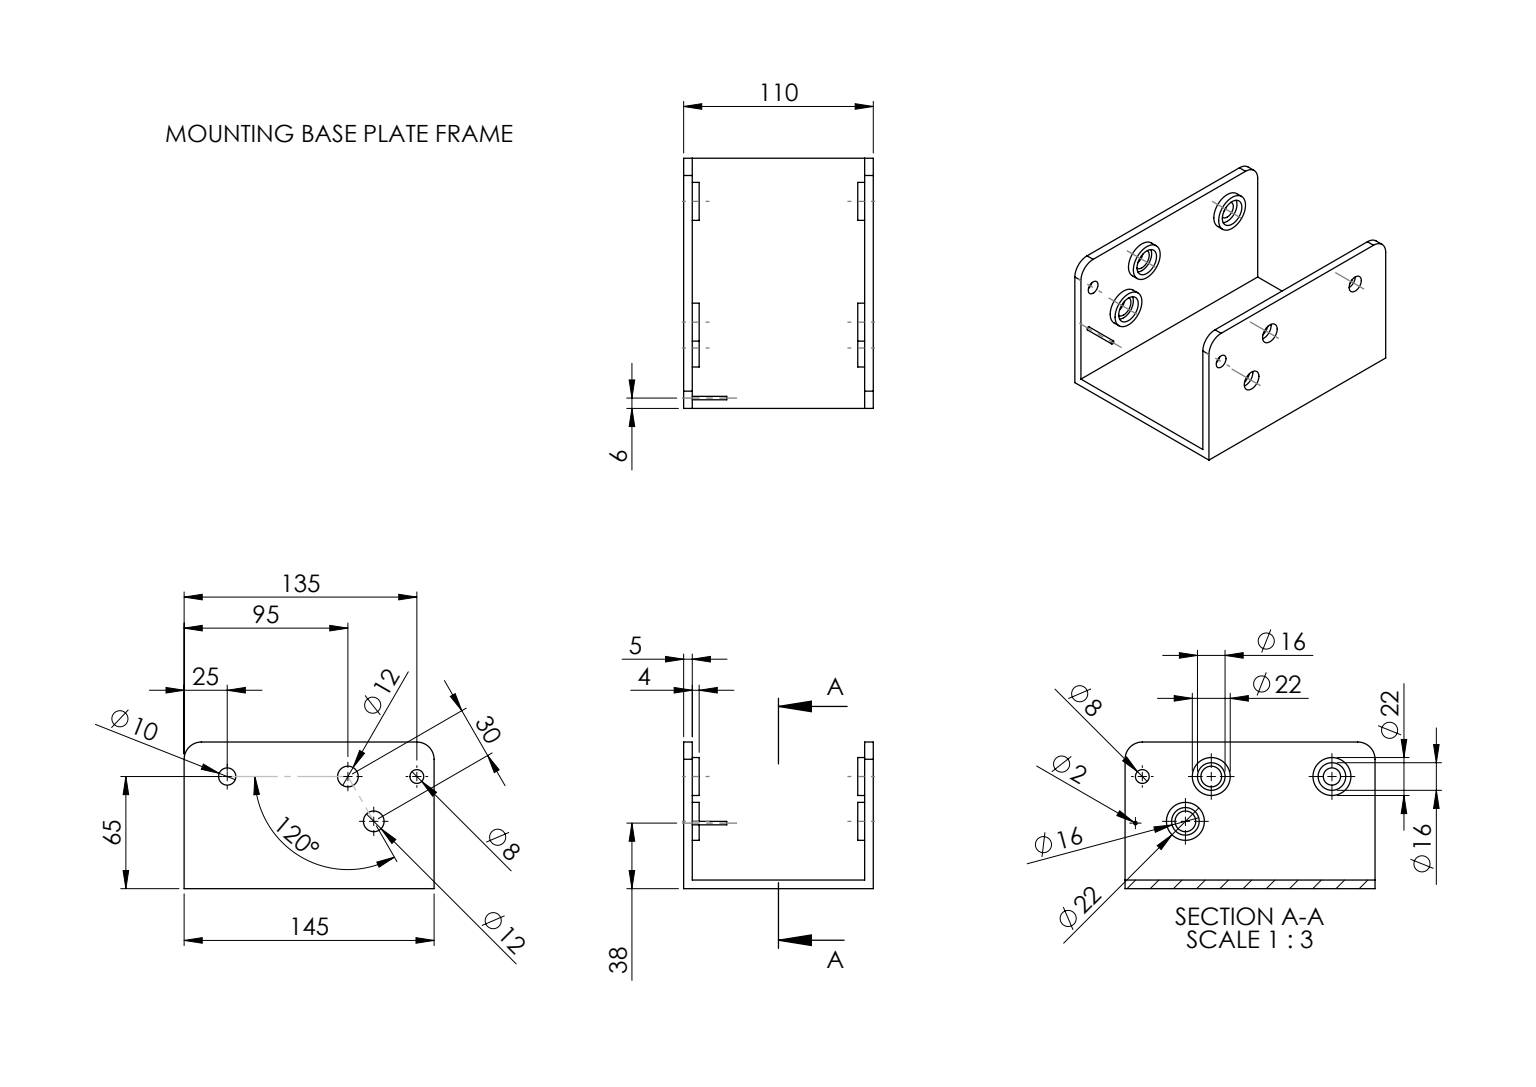
ISO-10303-21;
HEADER;
FILE_DESCRIPTION (('STEP AP214'),
    '1' );
FILE_NAME ('Mounting Base Plate Frame.step',
    '2026-09-28T15:49:00',
    ( '' ),
    ( '' ),
    'SwSTEP 2.0',
    'SolidWorks 2026',
    '' );
FILE_SCHEMA (( 'AUTOMOTIVE_DESIGN' ));
ENDSEC;

DATA;
#38=AXIS2_PLACEMENT_3D ( 'NONE', #16663, #5703, #35251 ) ;
#52=VERTEX_POINT ( 'NONE', #30421 ) ;
#68=CARTESIAN_POINT ( 'NONE',  ( -55.00000000000000000, -25.98076211353320275, 84.99999999999994316 ) ) ;
#85=CARTESIAN_POINT ( 'NONE',  ( -46.00000000000000000, 0.000000000000000000, 70.00000000000000000 ) ) ;
#102=EDGE_LOOP ( 'NONE', ( #28338, #13792, #13740, #22838 ) ) ;
#134=ORIENTED_EDGE ( 'NONE', *, *, #4280, .T. ) ;
#137=FACE_BOUND ( 'NONE', #21992, .T. ) ;
#175=CIRCLE ( 'NONE', #10540, 6.000000000000002665 ) ;
#195=DIRECTION ( 'NONE',  ( 1.000000000000000000, -0.000000000000000000, -0.000000000000000000 ) ) ;
#205=ORIENTED_EDGE ( 'NONE', *, *, #23774, .F. ) ;
#238=DIRECTION ( 'NONE',  ( 1.000000000000000000, -0.000000000000000000, -0.000000000000000000 ) ) ;
#239=ADVANCED_FACE ( 'NONE', ( #26385 ), #21143, .F. ) ;
#250=DIRECTION ( 'NONE',  ( 1.000000000000000000, -0.000000000000000000, -0.000000000000000000 ) ) ;
#253=CARTESIAN_POINT ( 'NONE',  ( 46.00000000000000000, 0.000000000000000000, 0.000000000000000000 ) ) ;
#269=EDGE_CURVE ( 'NONE', #16003, #16053, #12703, .T. ) ;
#279=FACE_OUTER_BOUND ( 'NONE', #7139, .T. ) ;
#299=DIRECTION ( 'NONE',  ( -1.000000000000000000, -0.000000000000000000, -0.000000000000000000 ) ) ;
#302=AXIS2_PLACEMENT_3D ( 'NONE', #13367, #4574, #23816 ) ;
#311=PLANE ( 'NONE',  #8495 ) ;
#330=CARTESIAN_POINT ( 'NONE',  ( 50.00000000000000000, 0.000000000000000000, 59.00000000000000000 ) ) ;
#339=DIRECTION ( 'NONE',  ( -1.000000000000000000, -1.734723475976807094E-16, 0.000000000000000000 ) ) ;
#344=CIRCLE ( 'NONE', #20442, 11.00000000000000000 ) ;
#406=CYLINDRICAL_SURFACE ( 'NONE', #13724, 5.000000000000011546 ) ;
#414=DIRECTION ( 'NONE',  ( -1.000000000000000000, -1.734723475976807094E-16, 0.000000000000000000 ) ) ;
#438=CARTESIAN_POINT ( 'NONE',  ( 50.00000000000000000, -25.98076211353320275, 95.99999999999991473 ) ) ;
#441=PLANE ( 'NONE',  #8977 ) ;
#443=CARTESIAN_POINT ( 'NONE',  ( 55.00000000000000000, 0.000000000000000000, 70.00000000000000000 ) ) ;
#461=FACE_BOUND ( 'NONE', #6076, .T. ) ;
#467=DIRECTION ( 'NONE',  ( 0.000000000000000000, -8.673617379884035472E-16, -1.000000000000000000 ) ) ;
#470=CARTESIAN_POINT ( 'NONE',  ( -55.00000000000000000, -25.98076211353320275, 78.99999999999992895 ) ) ;
#481=CIRCLE ( 'NONE', #21749, 8.000000000000007105 ) ;
#497=AXIS2_PLACEMENT_3D ( 'NONE', #3704, #28360, #7419 ) ;
#505=DIRECTION ( 'NONE',  ( -1.000000000000000000, -0.000000000000000000, -0.000000000000000000 ) ) ;
#525=FACE_BOUND ( 'NONE', #22321, .T. ) ;
#528=VECTOR ( 'NONE', #14611, 1000.000000000000000 ) ;
#536=ORIENTED_EDGE ( 'NONE', *, *, #30688, .F. ) ;
#546=EDGE_CURVE ( 'NONE', #32690, #18111, #21436, .T. ) ;
#564=FACE_OUTER_BOUND ( 'NONE', #12819, .T. ) ;
#566=AXIS2_PLACEMENT_3D ( 'NONE', #22239, #8555, #22407 ) ;
#568=DIRECTION ( 'NONE',  ( 0.000000000000000000, -1.000000000000000000, 0.000000000000000000 ) ) ;
#611=EDGE_LOOP ( 'NONE', ( #12181, #2390, #23196, #30546, #28877, #14877 ) ) ;
#616=CIRCLE ( 'NONE', #28227, 11.00000000000001066 ) ;
#622=VECTOR ( 'NONE', #10858, 1000.000000000000000 ) ;
#623=( GEOMETRIC_REPRESENTATION_CONTEXT ( 3 ) GLOBAL_UNCERTAINTY_ASSIGNED_CONTEXT ( ( #6706 ) ) GLOBAL_UNIT_ASSIGNED_CONTEXT ( ( #29466, #21700, #8019 ) ) REPRESENTATION_CONTEXT ( 'NONE', 'WORKASPACE' ) );
#624=AXIS2_PLACEMENT_3D ( 'NONE', #12818, #34782, #9575 ) ;
#651=EDGE_LOOP ( 'NONE', ( #4323, #22804, #11964, #18462 ) ) ;
#661=LINE ( 'NONE', #3396, #25418 ) ;
#676=CARTESIAN_POINT ( 'NONE',  ( -50.00000000000000000, 0.000000000000000000, 70.00000000000000000 ) ) ;
#678=EDGE_CURVE ( 'NONE', #10711, #10849, #15672, .T. ) ;
#788=EDGE_CURVE ( 'NONE', #2874, #30169, #31736, .T. ) ;
#810=ORIENTED_EDGE ( 'NONE', *, *, #8583, .F. ) ;
#835=CARTESIAN_POINT ( 'NONE',  ( 55.00000000000000000, -2.775557561562891351E-14, 106.0000000000000000 ) ) ;
#851=AXIS2_PLACEMENT_3D ( 'NONE', #33266, #6070, #8060 ) ;
#864=VERTEX_POINT ( 'NONE', #10853 ) ;
#873=LINE ( 'NONE', #25383, #15397 ) ;
#956=CIRCLE ( 'NONE', #18789, 11.00000000000000000 ) ;
#970=CARTESIAN_POINT ( 'NONE',  ( -55.00000000000000000, 19.99999999999998934, -25.00000000000000000 ) ) ;
#977=DIRECTION ( 'NONE',  ( 1.387778780781445922E-16, -1.000000000000000000, 0.000000000000000000 ) ) ;
#999=DIRECTION ( 'NONE',  ( 1.000000000000000000, -0.000000000000000000, -0.000000000000000000 ) ) ;
#1013=LINE ( 'NONE', #31248, #24550 ) ;
#1019=CARTESIAN_POINT ( 'NONE',  ( -46.00000000000000000, -25.98076211353320275, 84.99999999999992895 ) ) ;
#1024=PLANE ( 'NONE',  #11271 ) ;
#1030=EDGE_LOOP ( 'NONE', ( #7294, #134, #29404, #21726, #18517, #9971 ) ) ;
#1035=CARTESIAN_POINT ( 'NONE',  ( 50.00000000000000711, -2.775557561562891351E-14, 106.0000000000000000 ) ) ;
#1037=DIRECTION ( 'NONE',  ( -1.000000000000000000, -0.000000000000000000, -0.000000000000000000 ) ) ;
#1069=ORIENTED_EDGE ( 'NONE', *, *, #33286, .T. ) ;
#1080=CARTESIAN_POINT ( 'NONE',  ( 46.00000000000000000, -25.98076211353320275, 84.99999999999992895 ) ) ;
#1136=ADVANCED_FACE ( 'NONE', ( #19978 ), #5968, .T. ) ;
#1145=FACE_OUTER_BOUND ( 'NONE', #2016, .T. ) ;
#1156=ORIENTED_EDGE ( 'NONE', *, *, #678, .T. ) ;
#1193=DIRECTION ( 'NONE',  ( -1.000000000000000000, -1.734723475976807094E-16, 0.000000000000000000 ) ) ;
#1236=DIRECTION ( 'NONE',  ( 1.000000000000000000, -0.000000000000000000, -0.000000000000000000 ) ) ;
#1260=CARTESIAN_POINT ( 'NONE',  ( -50.00000000000000000, 0.000000000000000000, 70.00000000000000000 ) ) ;
#1297=AXIS2_PLACEMENT_3D ( 'NONE', #14046, #9000, #14227 ) ;
#1330=DIRECTION ( 'NONE',  ( 0.000000000000000000, 0.000000000000000000, 1.000000000000000000 ) ) ;
#1369=EDGE_CURVE ( 'NONE', #32690, #28784, #14777, .T. ) ;
#1398=AXIS2_PLACEMENT_3D ( 'NONE', #24633, #21379, #29506 ) ;
#1419=DIRECTION ( 'NONE',  ( -1.000000000000000000, -0.000000000000000000, -0.000000000000000000 ) ) ;
#1428=AXIS2_PLACEMENT_3D ( 'NONE', #32944, #339, #24842 ) ;
#1456=ORIENTED_EDGE ( 'NONE', *, *, #16234, .F. ) ;
#1495=CARTESIAN_POINT ( 'NONE',  ( 55.00000000000000000, 0.000000000000000000, 0.000000000000000000 ) ) ;
#1530=ADVANCED_FACE ( 'NONE', ( #4718, #7566 ), #29903, .F. ) ;
#1544=CYLINDRICAL_SURFACE ( 'NONE', #27428, 4.000000000000003553 ) ;
#1562=EDGE_LOOP ( 'NONE', ( #27042, #2895, #16503, #4140 ) ) ;
#1564=CYLINDRICAL_SURFACE ( 'NONE', #18869, 8.000000000000000000 ) ;
#1595=LINE ( 'NONE', #29140, #15472 ) ;
#1614=EDGE_CURVE ( 'NONE', #4202, #2870, #28977, .T. ) ;
#1635=VERTEX_POINT ( 'NONE', #13861 ) ;
#1646=CARTESIAN_POINT ( 'NONE',  ( -46.00000000000000000, -25.98076211353320275, 92.99999999999991473 ) ) ;
#1654=CARTESIAN_POINT ( 'NONE',  ( 55.00000000000000000, 0.000000000000000000, 64.00000000000000000 ) ) ;
#1719=AXIS2_PLACEMENT_3D ( 'NONE', #8421, #3401, #28059 ) ;
#1730=CARTESIAN_POINT ( 'NONE',  ( 50.00000000000000000, 20.00000000000001776, 120.0000000000000000 ) ) ;
#1738=ORIENTED_EDGE ( 'NONE', *, *, #29262, .T. ) ;
#1743=CARTESIAN_POINT ( 'NONE',  ( -46.00000000000000000, 0.000000000000000000, 0.000000000000000000 ) ) ;
#1769=FACE_OUTER_BOUND ( 'NONE', #102, .T. ) ;
#1794=LINE ( 'NONE', #5029, #30003 ) ;
#1800=DIRECTION ( 'NONE',  ( 1.000000000000000000, -0.000000000000000000, -0.000000000000000000 ) ) ;
#1803=CIRCLE ( 'NONE', #34001, 4.000000000000003553 ) ;
#1826=LINE ( 'NONE', #2496, #32565 ) ;
#1871=EDGE_CURVE ( 'NONE', #26262, #6240, #25561, .T. ) ;
#1899=CARTESIAN_POINT ( 'NONE',  ( -49.99999999999998579, -64.99999999999997158, 120.0000000000000000 ) ) ;
#1903=ORIENTED_EDGE ( 'NONE', *, *, #26827, .T. ) ;
#1910=CARTESIAN_POINT ( 'NONE',  ( -55.00000000000000000, 7.347880794884122694E-16, 76.00000000000001421 ) ) ;
#1912=ADVANCED_FACE ( 'NONE', ( #1962 ), #23923, .T. ) ;
#1919=ORIENTED_EDGE ( 'NONE', *, *, #34578, .F. ) ;
#1953=SURFACE_STYLE_FILL_AREA ( #20820 ) ;
#1962=FACE_OUTER_BOUND ( 'NONE', #32821, .T. ) ;
#1979=ORIENTED_EDGE ( 'NONE', *, *, #20002, .F. ) ;
#1992=VERTEX_POINT ( 'NONE', #32021 ) ;
#2000=EDGE_CURVE ( 'NONE', #6343, #26262, #18329, .T. ) ;
#2016=EDGE_LOOP ( 'NONE', ( #21254, #27790, #4374, #33130 ) ) ;
#2041=CYLINDRICAL_SURFACE ( 'NONE', #14651, 9.999999999999994671 ) ;
#2053=CARTESIAN_POINT ( 'NONE',  ( -46.00000000000000000, 0.000000000000000000, 0.000000000000000000 ) ) ;
#2057=ORIENTED_EDGE ( 'NONE', *, *, #7109, .T. ) ;
#2096=CARTESIAN_POINT ( 'NONE',  ( -55.00000000000000000, 19.99999999999998934, -15.00000000000001421 ) ) ;
#2099=CARTESIAN_POINT ( 'NONE',  ( -54.99999999999998579, -64.99999999999997158, 120.0000000000000000 ) ) ;
#2119=AXIS2_PLACEMENT_3D ( 'NONE', #20819, #4833, #23543 ) ;
#2188=AXIS2_PLACEMENT_3D ( 'NONE', #11595, #3159, #25470 ) ;
#2193=LINE ( 'NONE', #27017, #17471 ) ;
#2204=VERTEX_POINT ( 'NONE', #16506 ) ;
#2256=ORIENTED_EDGE ( 'NONE', *, *, #27606, .T. ) ;
#2260=EDGE_CURVE ( 'NONE', #17795, #35062, #21522, .T. ) ;
#2284=LINE ( 'NONE', #16455, #19273 ) ;
#2285=DIRECTION ( 'NONE',  ( 0.000000000000000000, 0.000000000000000000, -1.000000000000000000 ) ) ;
#2338=FACE_OUTER_BOUND ( 'NONE', #3922, .T. ) ;
#2385=CYLINDRICAL_SURFACE ( 'NONE', #21308, 6.000000000000005329 ) ;
#2390=ORIENTED_EDGE ( 'NONE', *, *, #3525, .T. ) ;
#2399=FACE_OUTER_BOUND ( 'NONE', #21454, .T. ) ;
#2410=PLANE ( 'NONE',  #29969 ) ;
#2454=CARTESIAN_POINT ( 'NONE',  ( 50.00000000000000711, 0.000000000000000000, -5.000000000000011546 ) ) ;
#2467=VERTEX_POINT ( 'NONE', #32694 ) ;
#2470=ORIENTED_EDGE ( 'NONE', *, *, #22024, .F. ) ;
#2496=CARTESIAN_POINT ( 'NONE',  ( -55.00000000000000000, 19.99999999999998934, 120.0000000000000000 ) ) ;
#2509=CARTESIAN_POINT ( 'NONE',  ( -50.00000000000000000, 19.99999999999998934, 120.0000000000000000 ) ) ;
#2533=DIRECTION ( 'NONE',  ( 0.000000000000000000, -1.000000000000000000, 0.000000000000000000 ) ) ;
#2539=VERTEX_POINT ( 'NONE', #32154 ) ;
#2562=ORIENTED_EDGE ( 'NONE', *, *, #10206, .T. ) ;
#2587=FACE_OUTER_BOUND ( 'NONE', #19208, .T. ) ;
#2612=AXIS2_PLACEMENT_3D ( 'NONE', #30286, #27413, #19276 ) ;
#2627=DIRECTION ( 'NONE',  ( 1.000000000000000000, -0.000000000000000000, -0.000000000000000000 ) ) ;
#2659=FACE_OUTER_BOUND ( 'NONE', #8842, .T. ) ;
#2708=LINE ( 'NONE', #29885, #33163 ) ;
#2739=DIRECTION ( 'NONE',  ( -1.000000000000000000, -0.000000000000000000, -0.000000000000000000 ) ) ;
#2767=VECTOR ( 'NONE', #22739, 1000.000000000000000 ) ;
#2773=LINE ( 'NONE', #13736, #622 ) ;
#2791=AXIS2_PLACEMENT_3D ( 'NONE', #4865, #10442, #16343 ) ;
#2811=LINE ( 'NONE', #13769, #21103 ) ;
#2823=FACE_OUTER_BOUND ( 'NONE', #6455, .T. ) ;
#2831=DIRECTION ( 'NONE',  ( 1.000000000000000000, -0.000000000000000000, -0.000000000000000000 ) ) ;
#2836=DIRECTION ( 'NONE',  ( 0.000000000000000000, -1.000000000000000000, 0.000000000000000000 ) ) ;
#2866=ADVANCED_FACE ( 'NONE', ( #9255 ), #14998, .F. ) ;
#2870=VERTEX_POINT ( 'NONE', #12310 ) ;
#2874=VERTEX_POINT ( 'NONE', #14639 ) ;
#2895=ORIENTED_EDGE ( 'NONE', *, *, #33936, .T. ) ;
#2911=FACE_BOUND ( 'NONE', #26913, .T. ) ;
#2932=AXIS2_PLACEMENT_3D ( 'NONE', #34706, #15585, #20808 ) ;
#2941=CARTESIAN_POINT ( 'NONE',  ( -55.00000000000000000, 19.99999999999998934, 120.0000000000000000 ) ) ;
#2963=CARTESIAN_POINT ( 'NONE',  ( 46.00000000000000000, 9.797174393178845379E-16, 78.00000000000001421 ) ) ;
#2964=CARTESIAN_POINT ( 'NONE',  ( -46.00000000000000000, 0.000000000000000000, 8.000000000000000000 ) ) ;
#3032=ORIENTED_EDGE ( 'NONE', *, *, #17647, .T. ) ;
#3042=CARTESIAN_POINT ( 'NONE',  ( 46.00000000000000000, 0.000000000000000000, 0.000000000000000000 ) ) ;
#3060=AXIS2_PLACEMENT_3D ( 'NONE', #18702, #24477, #4702 ) ;
#3102=EDGE_LOOP ( 'NONE', ( #5630, #4974, #16989, #17044 ) ) ;
#3106=DIRECTION ( 'NONE',  ( 1.000000000000000000, -0.000000000000000000, -0.000000000000000000 ) ) ;
#3122=EDGE_CURVE ( 'NONE', #18111, #31582, #15324, .T. ) ;
#3131=EDGE_CURVE ( 'NONE', #13387, #5141, #19671, .T. ) ;
#3150=CARTESIAN_POINT ( 'NONE',  ( -29.99999999999999645, -27.99999999999999289, 113.9999999999999858 ) ) ;
#3157=DIRECTION ( 'NONE',  ( 0.000000000000000000, 0.000000000000000000, 1.000000000000000000 ) ) ;
#3159=DIRECTION ( 'NONE',  ( -1.000000000000000000, -0.000000000000000000, -0.000000000000000000 ) ) ;
#3183=DIRECTION ( 'NONE',  ( -0.000000000000000000, 0.000000000000000000, -1.000000000000000000 ) ) ;
#3201=DIRECTION ( 'NONE',  ( -1.000000000000000000, -0.000000000000000000, -0.000000000000000000 ) ) ;
#3208=AXIS2_PLACEMENT_3D ( 'NONE', #85, #33034, #11072 ) ;
#3213=ORIENTED_EDGE ( 'NONE', *, *, #18521, .F. ) ;
#3216=LINE ( 'NONE', #6601, #21447 ) ;
#3253=DIRECTION ( 'NONE',  ( 0.000000000000000000, 0.000000000000000000, 1.000000000000000000 ) ) ;
#3254=PLANE ( 'NONE',  #8668 ) ;
#3267=AXIS2_PLACEMENT_3D ( 'NONE', #20064, #28369, #6398 ) ;
#3309=VERTEX_POINT ( 'NONE', #13194 ) ;
#3324=ORIENTED_EDGE ( 'NONE', *, *, #1369, .T. ) ;
#3332=CARTESIAN_POINT ( 'NONE',  ( -50.00000000000000000, 19.99999999999998934, 120.0000000000000000 ) ) ;
#3396=CARTESIAN_POINT ( 'NONE',  ( 0.000000000000000000, 10.00000000000000888, -25.00000000000000000 ) ) ;
#3401=DIRECTION ( 'NONE',  ( 1.000000000000000000, 1.734723475976807094E-16, -0.000000000000000000 ) ) ;
#3426=ORIENTED_EDGE ( 'NONE', *, *, #17908, .F. ) ;
#3429=EDGE_CURVE ( 'NONE', #21242, #33174, #16803, .T. ) ;
#3449=CIRCLE ( 'NONE', #1719, 0.9999999999999974465 ) ;
#3475=CIRCLE ( 'NONE', #18979, 8.000000000000000000 ) ;
#3494=DIRECTION ( 'NONE',  ( -0.000000000000000000, 0.000000000000000000, 1.000000000000000000 ) ) ;
#3504=FACE_BOUND ( 'NONE', #23755, .T. ) ;
#3525=EDGE_CURVE ( 'NONE', #26450, #35140, #7631, .T. ) ;
#3592=EDGE_CURVE ( 'NONE', #6257, #21944, #34213, .T. ) ;
#3595=DIRECTION ( 'NONE',  ( 1.000000000000000000, -0.000000000000000000, -0.000000000000000000 ) ) ;
#3598=EDGE_LOOP ( 'NONE', ( #31397, #23988, #13480, #29011 ) ) ;
#3620=LINE ( 'NONE', #22670, #21125 ) ;
#3637=CARTESIAN_POINT ( 'NONE',  ( -50.00000000000000000, 0.000000000000000000, -5.000000000000011546 ) ) ;
#3646=VECTOR ( 'NONE', #26534, 1000.000000000000000 ) ;
#3655=ORIENTED_EDGE ( 'NONE', *, *, #29996, .T. ) ;
#3670=APPLICATION_CONTEXT ( 'automotive_design' ) ;
#3680=DIRECTION ( 'NONE',  ( -1.734723475976807094E-16, 1.000000000000000000, 0.000000000000000000 ) ) ;
#3704=CARTESIAN_POINT ( 'NONE',  ( -50.00000000000000000, 0.000000000000000000, 70.00000000000000000 ) ) ;
#3743=EDGE_LOOP ( 'NONE', ( #1903, #25067 ) ) ;
#3744=DIRECTION ( 'NONE',  ( -1.000000000000000000, 0.000000000000000000, 0.000000000000000000 ) ) ;
#3759=FACE_OUTER_BOUND ( 'NONE', #5965, .T. ) ;
#3797=CARTESIAN_POINT ( 'NONE',  ( -29.99999999999999645, -27.99999999999999289, 113.9999999999999858 ) ) ;
#3828=DIRECTION ( 'NONE',  ( 1.000000000000000000, 1.734723475976807094E-16, -0.000000000000000000 ) ) ;
#3829=EDGE_CURVE ( 'NONE', #2870, #4202, #18567, .T. ) ;
#3857=EDGE_CURVE ( 'NONE', #15308, #17487, #9359, .T. ) ;
#3864=DIRECTION ( 'NONE',  ( -1.000000000000000000, -0.000000000000000000, -0.000000000000000000 ) ) ;
#3869=ORIENTED_EDGE ( 'NONE', *, *, #12177, .T. ) ;
#3877=VERTEX_POINT ( 'NONE', #8076 ) ;
#3880=CIRCLE ( 'NONE', #7307, 6.000000000000005329 ) ;
#3901=CARTESIAN_POINT ( 'NONE',  ( -50.00000000000000000, 10.00000000000000888, 120.0000000000000000 ) ) ;
#3906=CARTESIAN_POINT ( 'NONE',  ( -46.00000000000000000, 0.000000000000000000, 0.000000000000000000 ) ) ;
#3922=EDGE_LOOP ( 'NONE', ( #7495, #30740, #14943, #6320 ) ) ;
#3934=AXIS2_PLACEMENT_3D ( 'NONE', #1260, #31326, #28984 ) ;
#4017=ORIENTED_EDGE ( 'NONE', *, *, #14512, .T. ) ;
#4095=FACE_OUTER_BOUND ( 'NONE', #13543, .T. ) ;
#4096=ORIENTED_EDGE ( 'NONE', *, *, #7699, .F. ) ;
#4103=CIRCLE ( 'NONE', #624, 0.9999999999999974465 ) ;
#4104=LINE ( 'NONE', #18469, #31061 ) ;
#4140=ORIENTED_EDGE ( 'NONE', *, *, #17735, .F. ) ;
#4184=DIRECTION ( 'NONE',  ( -1.000000000000000000, -1.734723475976807094E-16, 0.000000000000000000 ) ) ;
#4189=DIRECTION ( 'NONE',  ( 1.387778780781445922E-16, -1.000000000000000000, 0.000000000000000000 ) ) ;
#4202=VERTEX_POINT ( 'NONE', #33997 ) ;
#4208=ADVANCED_FACE ( 'NONE', ( #13972, #6046, #32712, #19698, #2659 ), #32888, .T. ) ;
#4212=CYLINDRICAL_SURFACE ( 'NONE', #27884, 8.000000000000007105 ) ;
#4215=CYLINDRICAL_SURFACE ( 'NONE', #24885, 6.000000000000005329 ) ;
#4239=ADVANCED_FACE ( 'NONE', ( #19021, #14312 ), #28018, .F. ) ;
#4240=DIRECTION ( 'NONE',  ( 0.000000000000000000, 0.000000000000000000, -1.000000000000000000 ) ) ;
#4280=EDGE_CURVE ( 'NONE', #30634, #22786, #19147, .T. ) ;
#4288=CARTESIAN_POINT ( 'NONE',  ( -46.00000000000000000, 0.000000000000000000, 78.00000000000001421 ) ) ;
#4303=VERTEX_POINT ( 'NONE', #16299 ) ;
#4309=ORIENTED_EDGE ( 'NONE', *, *, #34176, .F. ) ;
#4310=EDGE_CURVE ( 'NONE', #5141, #28364, #11449, .T. ) ;
#4323=ORIENTED_EDGE ( 'NONE', *, *, #1614, .F. ) ;
#4356=ORIENTED_EDGE ( 'NONE', *, *, #18073, .F. ) ;
#4374=ORIENTED_EDGE ( 'NONE', *, *, #18934, .F. ) ;
#4448=ORIENTED_EDGE ( 'NONE', *, *, #18732, .F. ) ;
#4457=ADVANCED_FACE ( 'NONE', ( #19876 ), #28545, .T. ) ;
#4470=ORIENTED_EDGE ( 'NONE', *, *, #20316, .T. ) ;
#4485=AXIS2_PLACEMENT_3D ( 'NONE', #29986, #5324, #24932 ) ;
#4491=DIRECTION ( 'NONE',  ( 1.000000000000000000, -0.000000000000000000, -0.000000000000000000 ) ) ;
#4519=DIRECTION ( 'NONE',  ( 1.000000000000000000, -0.000000000000000000, -0.000000000000000000 ) ) ;
#4535=CARTESIAN_POINT ( 'NONE',  ( 50.00000000000000000, 20.00000000000001776, -25.00000000000000000 ) ) ;
#4545=DIRECTION ( 'NONE',  ( -1.000000000000000000, -0.000000000000000000, -0.000000000000000000 ) ) ;
#4546=EDGE_LOOP ( 'NONE', ( #17373, #23327 ) ) ;
#4574=DIRECTION ( 'NONE',  ( 1.000000000000000000, 0.000000000000000000, 0.000000000000000000 ) ) ;
#4595=VECTOR ( 'NONE', #4519, 1000.000000000000000 ) ;
#4598=EDGE_LOOP ( 'NONE', ( #18366, #4470 ) ) ;
#4616=CARTESIAN_POINT ( 'NONE',  ( -49.99999999999998579, -64.99999999999997158, -25.00000000000000000 ) ) ;
#4620=LINE ( 'NONE', #1910, #35481 ) ;
#4627=CARTESIAN_POINT ( 'NONE',  ( -50.00000000000000000, 19.99999999999998934, 120.0000000000000000 ) ) ;
#4641=VECTOR ( 'NONE', #20780, 1000.000000000000000 ) ;
#4646=EDGE_LOOP ( 'NONE', ( #12462, #23064 ) ) ;
#4683=CARTESIAN_POINT ( 'NONE',  ( -29.99999999999999645, -26.99999999999999645, 113.9999999999999858 ) ) ;
#4702=DIRECTION ( 'NONE',  ( 0.000000000000000000, 0.000000000000000000, 1.000000000000000000 ) ) ;
#4718=FACE_BOUND ( 'NONE', #4546, .T. ) ;
#4721=AXIS2_PLACEMENT_3D ( 'NONE', #25348, #5898, #22098 ) ;
#4770=FACE_OUTER_BOUND ( 'NONE', #28713, .T. ) ;
#4772=ORIENTED_EDGE ( 'NONE', *, *, #31314, .F. ) ;
#4788=LINE ( 'NONE', #4616, #35231 ) ;
#4808=ORIENTED_EDGE ( 'NONE', *, *, #3131, .T. ) ;
#4833=DIRECTION ( 'NONE',  ( -1.000000000000000000, -1.734723475976807094E-16, -0.000000000000000000 ) ) ;
#4839=VERTEX_POINT ( 'NONE', #11889 ) ;
#4857=AXIS2_PLACEMENT_3D ( 'NONE', #9340, #1419, #20124 ) ;
#4861=ORIENTED_EDGE ( 'NONE', *, *, #15180, .T. ) ;
#4865=CARTESIAN_POINT ( 'NONE',  ( 46.00000000000000000, 0.000000000000000000, 70.00000000000000000 ) ) ;
#4889=ORIENTED_EDGE ( 'NONE', *, *, #7647, .T. ) ;
#4974=ORIENTED_EDGE ( 'NONE', *, *, #3829, .F. ) ;
#4985=CIRCLE ( 'NONE', #9573, 10.00000000000000000 ) ;
#5003=CARTESIAN_POINT ( 'NONE',  ( -46.00000000000000000, 1.347111479062088405E-15, -11.00000000000000000 ) ) ;
#5007=CIRCLE ( 'NONE', #10193, 6.000000000000005329 ) ;
#5015=CIRCLE ( 'NONE', #9027, 4.000000000000006217 ) ;
#5029=CARTESIAN_POINT ( 'NONE',  ( -55.00000000000000000, 10.00000000000000888, 120.0000000000000000 ) ) ;
#5035=LINE ( 'NONE', #35454, #33534 ) ;
#5039=CIRCLE ( 'NONE', #9624, 4.000000000000003553 ) ;
#5044=EDGE_CURVE ( 'NONE', #11158, #11697, #2193, .T. ) ;
#5106=AXIS2_PLACEMENT_3D ( 'NONE', #16854, #3201, #30908 ) ;
#5110=CARTESIAN_POINT ( 'NONE',  ( -50.00000000000000000, 0.000000000000000000, 0.000000000000000000 ) ) ;
#5124=ORIENTED_EDGE ( 'NONE', *, *, #9438, .F. ) ;
#5139=CARTESIAN_POINT ( 'NONE',  ( -55.00000000000000000, -2.775557561562891351E-14, 110.0000000000000000 ) ) ;
#5141=VERTEX_POINT ( 'NONE', #32054 ) ;
#5166=SHAPE_REPRESENTATION_RELATIONSHIP ( 'NONE' , 'NONE' ,  #13971, #12087 ) ;
#5198=LINE ( 'NONE', #1646, #8429 ) ;
#5203=ORIENTED_EDGE ( 'NONE', *, *, #9976, .F. ) ;
#5226=FACE_OUTER_BOUND ( 'NONE', #23693, .T. ) ;
#5251=EDGE_LOOP ( 'NONE', ( #31104, #6666, #24073, #34586 ) ) ;
#5260=VERTEX_POINT ( 'NONE', #5917 ) ;
#5324=DIRECTION ( 'NONE',  ( -1.000000000000000000, -0.000000000000000000, 0.000000000000000000 ) ) ;
#5341=ORIENTED_EDGE ( 'NONE', *, *, #27641, .F. ) ;
#5348=AXIS2_PLACEMENT_3D ( 'NONE', #1495, #20913, #31381 ) ;
#5350=AXIS2_PLACEMENT_3D ( 'NONE', #17684, #18216, #29222 ) ;
#5364=LINE ( 'NONE', #8220, #31414 ) ;
#5378=ADVANCED_FACE ( 'NONE', ( #3759 ), #6803, .F. ) ;
#5390=ORIENTED_EDGE ( 'NONE', *, *, #7142, .F. ) ;
#5494=AXIS2_PLACEMENT_3D ( 'NONE', #33073, #19372, #11280 ) ;
#5519=DIRECTION ( 'NONE',  ( -1.000000000000000000, 0.000000000000000000, 0.000000000000000000 ) ) ;
#5551=DIRECTION ( 'NONE',  ( -1.000000000000000000, -0.000000000000000000, -0.000000000000000000 ) ) ;
#5555=DIRECTION ( 'NONE',  ( 0.000000000000000000, 0.000000000000000000, -1.000000000000000000 ) ) ;
#5560=DIRECTION ( 'NONE',  ( -1.000000000000000000, -0.000000000000000000, 0.000000000000000000 ) ) ;
#5628=CARTESIAN_POINT ( 'NONE',  ( -50.00000000000000000, 19.99999999999998934, -25.00000000000000000 ) ) ;
#5630=ORIENTED_EDGE ( 'NONE', *, *, #8997, .F. ) ;
#5635=DIRECTION ( 'NONE',  ( -1.000000000000000000, 0.000000000000000000, -0.000000000000000000 ) ) ;
#5672=CYLINDRICAL_SURFACE ( 'NONE', #11817, 8.000000000000000000 ) ;
#5694=LINE ( 'NONE', #31059, #6868 ) ;
#5703=DIRECTION ( 'NONE',  ( -1.000000000000000000, 0.000000000000000000, 0.000000000000000000 ) ) ;
#5731=ORIENTED_EDGE ( 'NONE', *, *, #28822, .T. ) ;
#5745=ORIENTED_EDGE ( 'NONE', *, *, #17445, .F. ) ;
#5817=EDGE_CURVE ( 'NONE', #26586, #31687, #11215, .T. ) ;
#5850=DIRECTION ( 'NONE',  ( 0.000000000000000000, 0.000000000000000000, -1.000000000000000000 ) ) ;
#5884=VERTEX_POINT ( 'NONE', #31429 ) ;
#5892=EDGE_LOOP ( 'NONE', ( #19435, #22716, #25356, #12042 ) ) ;
#5898=DIRECTION ( 'NONE',  ( -1.000000000000000000, -0.000000000000000000, -0.000000000000000000 ) ) ;
#5904=CARTESIAN_POINT ( 'NONE',  ( -50.00000000000000000, 0.000000000000000000, 0.000000000000000000 ) ) ;
#5917=CARTESIAN_POINT ( 'NONE',  ( 55.00000000000000000, -2.726571689596996976E-14, 114.0000000000000000 ) ) ;
#5965=EDGE_LOOP ( 'NONE', ( #27239, #30604, #8467, #7486 ) ) ;
#5968=CYLINDRICAL_SURFACE ( 'NONE', #31821, 11.00000000000000000 ) ;
#5982=FACE_OUTER_BOUND ( 'NONE', #23235, .T. ) ;
#6008=ORIENTED_EDGE ( 'NONE', *, *, #14512, .F. ) ;
#6015=CARTESIAN_POINT ( 'NONE',  ( -50.00000000000000000, -25.98076211353320275, 73.99999999999992895 ) ) ;
#6040=FACE_BOUND ( 'NONE', #4646, .T. ) ;
#6046=FACE_BOUND ( 'NONE', #24144, .T. ) ;
#6055=CARTESIAN_POINT ( 'NONE',  ( -55.00000000000000000, 10.00000000000000888, 110.0000000000000000 ) ) ;
#6068=ORIENTED_EDGE ( 'NONE', *, *, #1614, .T. ) ;
#6070=DIRECTION ( 'NONE',  ( 1.000000000000000000, 1.734723475976807094E-16, 0.000000000000000000 ) ) ;
#6076=EDGE_LOOP ( 'NONE', ( #9789, #27808 ) ) ;
#6086=CARTESIAN_POINT ( 'NONE',  ( 46.00000000000000000, -25.98076211353320275, 84.99999999999992895 ) ) ;
#6167=CARTESIAN_POINT ( 'NONE',  ( 50.00000000000000000, 20.00000000000001776, 110.0000000000000000 ) ) ;
#6168=EDGE_CURVE ( 'NONE', #7646, #22338, #7296, .T. ) ;
#6187=FACE_BOUND ( 'NONE', #11736, .T. ) ;
#6189=DIRECTION ( 'NONE',  ( 0.000000000000000000, 1.000000000000000000, 0.000000000000000000 ) ) ;
#6196=PLANE ( 'NONE',  #25071 ) ;
#6198=ADVANCED_FACE ( 'NONE', ( #16090, #27108 ), #26392, .F. ) ;
#6201=FACE_BOUND ( 'NONE', #13504, .T. ) ;
#6204=ORIENTED_EDGE ( 'NONE', *, *, #6168, .T. ) ;
#6240=VERTEX_POINT ( 'NONE', #6015 ) ;
#6241=ORIENTED_EDGE ( 'NONE', *, *, #22646, .F. ) ;
#6244=ADVANCED_FACE ( 'NONE', ( #8176 ), #5672, .F. ) ;
#6255=DIRECTION ( 'NONE',  ( 0.000000000000000000, 0.000000000000000000, 1.000000000000000000 ) ) ;
#6257=VERTEX_POINT ( 'NONE', #3150 ) ;
#6263=PLANE ( 'NONE',  #25922 ) ;
#6288=( GEOMETRIC_REPRESENTATION_CONTEXT ( 3 ) GLOBAL_UNCERTAINTY_ASSIGNED_CONTEXT ( ( #20405 ) ) GLOBAL_UNIT_ASSIGNED_CONTEXT ( ( #18133, #24101, #7159 ) ) REPRESENTATION_CONTEXT ( 'NONE', 'WORKASPACE' ) );
#6298=DIRECTION ( 'NONE',  ( -1.000000000000000000, 0.000000000000000000, 0.000000000000000000 ) ) ;
#6320=ORIENTED_EDGE ( 'NONE', *, *, #23648, .F. ) ;
#6343=VERTEX_POINT ( 'NONE', #24759 ) ;
#6360=ORIENTED_EDGE ( 'NONE', *, *, #29391, .F. ) ;
#6398=DIRECTION ( 'NONE',  ( 0.000000000000000000, 0.000000000000000000, -1.000000000000000000 ) ) ;
#6431=CARTESIAN_POINT ( 'NONE',  ( -55.00000000000000000, -2.775557561562891351E-14, 106.0000000000000000 ) ) ;
#6435=FACE_OUTER_BOUND ( 'NONE', #6469, .T. ) ;
#6455=EDGE_LOOP ( 'NONE', ( #8898, #4356 ) ) ;
#6459=ORIENTED_EDGE ( 'NONE', *, *, #29262, .F. ) ;
#6469=EDGE_LOOP ( 'NONE', ( #11084, #10812 ) ) ;
#6507=DIRECTION ( 'NONE',  ( 1.000000000000000000, 1.387778780781445922E-16, 0.000000000000000000 ) ) ;
#6534=CARTESIAN_POINT ( 'NONE',  ( -55.00000000000000000, 19.99999999999998934, -15.00000000000001421 ) ) ;
#6538=LINE ( 'NONE', #28512, #26808 ) ;
#6541=EDGE_LOOP ( 'NONE', ( #26232, #26171, #9011, #1156 ) ) ;
#6601=CARTESIAN_POINT ( 'NONE',  ( 46.00000000000000000, 0.000000000000000000, 59.00000000000000000 ) ) ;
#6643=DIRECTION ( 'NONE',  ( 0.000000000000000000, 0.000000000000000000, -1.000000000000000000 ) ) ;
#6659=EDGE_CURVE ( 'NONE', #6941, #2467, #8961, .T. ) ;
#6666=ORIENTED_EDGE ( 'NONE', *, *, #3131, .F. ) ;
#6673=EDGE_LOOP ( 'NONE', ( #6459, #28530, #2256, #34420 ) ) ;
#6706=UNCERTAINTY_MEASURE_WITH_UNIT (LENGTH_MEASURE( 1.000000000000000082E-05 ), #29466, 'distance_accuracy_value', 'NONE');
#6715=AXIS2_PLACEMENT_3D ( 'NONE', #22348, #33343, #568 ) ;
#6776=ORIENTED_EDGE ( 'NONE', *, *, #11610, .T. ) ;
#6777=CIRCLE ( 'NONE', #11388, 6.000000000000005329 ) ;
#6780=DIRECTION ( 'NONE',  ( -1.000000000000000000, -0.000000000000000000, -0.000000000000000000 ) ) ;
#6803=CYLINDRICAL_SURFACE ( 'NONE', #22103, 4.000000000000003553 ) ;
#6821=DIRECTION ( 'NONE',  ( -1.000000000000000000, -0.000000000000000000, -0.000000000000000000 ) ) ;
#6828=ORIENTED_EDGE ( 'NONE', *, *, #26966, .T. ) ;
#6836=AXIS2_PLACEMENT_3D ( 'NONE', #22756, #28002, #33754 ) ;
#6843=ORIENTED_EDGE ( 'NONE', *, *, #21312, .T. ) ;
#6867=FACE_OUTER_BOUND ( 'NONE', #11907, .T. ) ;
#6868=VECTOR ( 'NONE', #999, 1000.000000000000000 ) ;
#6891=DIRECTION ( 'NONE',  ( 0.000000000000000000, 0.000000000000000000, -1.000000000000000000 ) ) ;
#6936=FACE_OUTER_BOUND ( 'NONE', #21499, .T. ) ;
#6941=VERTEX_POINT ( 'NONE', #3637 ) ;
#6957=CARTESIAN_POINT ( 'NONE',  ( 50.00000000000000711, 7.347880794884119736E-16, 76.00000000000001421 ) ) ;
#6965=CARTESIAN_POINT ( 'NONE',  ( 55.00000000000000000, 7.347880794884119736E-16, 76.00000000000001421 ) ) ;
#6990=ORIENTED_EDGE ( 'NONE', *, *, #27868, .T. ) ;
#7024=VECTOR ( 'NONE', #26418, 1000.000000000000000 ) ;
#7069=ADVANCED_FACE ( 'NONE', ( #35431 ), #21535, .F. ) ;
#7097=CARTESIAN_POINT ( 'NONE',  ( 55.00000000000000000, 0.000000000000000000, 0.000000000000000000 ) ) ;
#7098=EDGE_CURVE ( 'NONE', #33174, #21242, #27422, .T. ) ;
#7109=EDGE_CURVE ( 'NONE', #23379, #28580, #5198, .T. ) ;
#7125=DIRECTION ( 'NONE',  ( 0.000000000000000000, -1.000000000000000000, 0.000000000000000000 ) ) ;
#7134=DIRECTION ( 'NONE',  ( -1.000000000000000000, 0.000000000000000000, 0.000000000000000000 ) ) ;
#7139=EDGE_LOOP ( 'NONE', ( #28135, #14330 ) ) ;
#7140=CARTESIAN_POINT ( 'NONE',  ( 46.00000000000000000, 1.347111479062090180E-15, 81.00000000000001421 ) ) ;
#7142=EDGE_CURVE ( 'NONE', #26801, #24996, #1826, .T. ) ;
#7143=ORIENTED_EDGE ( 'NONE', *, *, #9438, .T. ) ;
#7146=DIRECTION ( 'NONE',  ( 0.000000000000000000, 0.000000000000000000, -1.000000000000000000 ) ) ;
#7159=( NAMED_UNIT ( * ) SI_UNIT ( $, .STERADIAN. ) SOLID_ANGLE_UNIT ( ) );
#7225=PRODUCT_DEFINITION_SHAPE ( 'NONE', 'NONE',  #33925 ) ;
#7252=LINE ( 'NONE', #12852, #18227 ) ;
#7284=VECTOR ( 'NONE', #12162, 1000.000000000000000 ) ;
#7290=CARTESIAN_POINT ( 'NONE',  ( -55.00000000000000000, -2.775557561562891351E-14, 106.0000000000000000 ) ) ;
#7294=ORIENTED_EDGE ( 'NONE', *, *, #18679, .T. ) ;
#7296=LINE ( 'NONE', #18451, #30240 ) ;
#7307=AXIS2_PLACEMENT_3D ( 'NONE', #68, #18971, #32473 ) ;
#7317=ORIENTED_EDGE ( 'NONE', *, *, #20316, .F. ) ;
#7373=CYLINDRICAL_SURFACE ( 'NONE', #11088, 6.000000000000005329 ) ;
#7419=DIRECTION ( 'NONE',  ( 0.000000000000000000, -1.000000000000000000, 0.000000000000000000 ) ) ;
#7458=AXIS2_PLACEMENT_3D ( 'NONE', #29527, #7893, #21223 ) ;
#7478=CARTESIAN_POINT ( 'NONE',  ( 50.00000000000000711, 0.000000000000000000, 70.00000000000000000 ) ) ;
#7486=ORIENTED_EDGE ( 'NONE', *, *, #22024, .T. ) ;
#7495=ORIENTED_EDGE ( 'NONE', *, *, #15610, .F. ) ;
#7499=DIRECTION ( 'NONE',  ( 1.000000000000000000, 0.000000000000000000, 0.000000000000000000 ) ) ;
#7517=AXIS2_PLACEMENT_3D ( 'NONE', #16405, #16594, #13551 ) ;
#7531=ORIENTED_EDGE ( 'NONE', *, *, #13427, .T. ) ;
#7535=EDGE_CURVE ( 'NONE', #5141, #13387, #3880, .T. ) ;
#7566=FACE_OUTER_BOUND ( 'NONE', #29465, .T. ) ;
#7582=ADVANCED_FACE ( 'NONE', ( #35029 ), #8689, .F. ) ;
#7592=DIRECTION ( 'NONE',  ( 0.000000000000000000, 0.000000000000000000, -1.000000000000000000 ) ) ;
#7593=DIRECTION ( 'NONE',  ( 0.000000000000000000, 0.000000000000000000, 1.000000000000000000 ) ) ;
#7595=LINE ( 'NONE', #5628, #19510 ) ;
#7600=DIRECTION ( 'NONE',  ( -1.000000000000000000, -1.734723475976807094E-16, 0.000000000000000000 ) ) ;
#7631=CIRCLE ( 'NONE', #14506, 10.00000000000000000 ) ;
#7639=ORIENTED_EDGE ( 'NONE', *, *, #35571, .T. ) ;
#7646=VERTEX_POINT ( 'NONE', #2964 ) ;
#7647=EDGE_CURVE ( 'NONE', #28364, #4303, #5007, .T. ) ;
#7657=SURFACE_STYLE_USAGE ( .BOTH. , #32504 ) ;
#7683=DIRECTION ( 'NONE',  ( 0.000000000000000000, 0.000000000000000000, 1.000000000000000000 ) ) ;
#7697=EDGE_CURVE ( 'NONE', #30988, #33867, #15331, .T. ) ;
#7699=EDGE_CURVE ( 'NONE', #26586, #17467, #22369, .T. ) ;
#7701=EDGE_CURVE ( 'NONE', #31687, #30036, #27964, .T. ) ;
#7707=VECTOR ( 'NONE', #16321, 1000.000000000000000 ) ;
#7709=DIRECTION ( 'NONE',  ( 0.000000000000000000, 0.000000000000000000, -1.000000000000000000 ) ) ;
#7719=DIRECTION ( 'NONE',  ( 0.000000000000000000, 0.000000000000000000, 1.000000000000000000 ) ) ;
#7734=ORIENTED_EDGE ( 'NONE', *, *, #32780, .T. ) ;
#7735=ORIENTED_EDGE ( 'NONE', *, *, #13477, .T. ) ;
#7741=EDGE_CURVE ( 'NONE', #31582, #16323, #19918, .T. ) ;
#7752=CIRCLE ( 'NONE', #302, 6.000000000000005329 ) ;
#7780=DIRECTION ( 'NONE',  ( 0.000000000000000000, 1.000000000000000000, 0.000000000000000000 ) ) ;
#7794=AXIS2_PLACEMENT_3D ( 'NONE', #24403, #19162, #33215 ) ;
#7840=CARTESIAN_POINT ( 'NONE',  ( -55.00000000000000000, -25.98076211353320275, 84.99999999999994316 ) ) ;
#7846=ORIENTED_EDGE ( 'NONE', *, *, #13477, .F. ) ;
#7864=DIRECTION ( 'NONE',  ( -1.000000000000000000, -0.000000000000000000, -0.000000000000000000 ) ) ;
#7878=CIRCLE ( 'NONE', #33203, 11.00000000000001066 ) ;
#7893=DIRECTION ( 'NONE',  ( 1.000000000000000000, -0.000000000000000000, -0.000000000000000000 ) ) ;
#7925=ORIENTED_EDGE ( 'NONE', *, *, #26088, .T. ) ;
#7960=ORIENTED_EDGE ( 'NONE', *, *, #34015, .T. ) ;
#7972=ORIENTED_EDGE ( 'NONE', *, *, #13407, .F. ) ;
#7980=AXIS2_PLACEMENT_3D ( 'NONE', #28486, #25970, #25802 ) ;
#8019=( NAMED_UNIT ( * ) SI_UNIT ( $, .STERADIAN. ) SOLID_ANGLE_UNIT ( ) );
#8022=DIRECTION ( 'NONE',  ( 0.000000000000000000, 0.000000000000000000, -1.000000000000000000 ) ) ;
#8035=DIRECTION ( 'NONE',  ( 0.000000000000000000, 0.000000000000000000, -1.000000000000000000 ) ) ;
#8050=DIRECTION ( 'NONE',  ( 0.000000000000000000, 0.000000000000000000, 1.000000000000000000 ) ) ;
#8060=DIRECTION ( 'NONE',  ( -1.734723475976807094E-16, 1.000000000000000000, 0.000000000000000000 ) ) ;
#8065=EDGE_LOOP ( 'NONE', ( #4448, #10738 ) ) ;
#8076=CARTESIAN_POINT ( 'NONE',  ( 50.00000000000000000, -59.99999999999997158, -25.00000000000000000 ) ) ;
#8080=DIRECTION ( 'NONE',  ( 1.000000000000000000, -0.000000000000000000, -0.000000000000000000 ) ) ;
#8088=ORIENTED_EDGE ( 'NONE', *, *, #31543, .T. ) ;
#8095=CIRCLE ( 'NONE', #12711, 4.000000000000003553 ) ;
#8176=FACE_OUTER_BOUND ( 'NONE', #18389, .T. ) ;
#8211=LINE ( 'NONE', #19189, #14522 ) ;
#8220=CARTESIAN_POINT ( 'NONE',  ( -46.00000000000000000, -25.98076211353320275, 73.99999999999992895 ) ) ;
#8227=ORIENTED_EDGE ( 'NONE', *, *, #22056, .T. ) ;
#8237=ADVANCED_FACE ( 'NONE', ( #11884 ), #20684, .F. ) ;
#8265=PLANE ( 'NONE',  #1428 ) ;
#8272=ORIENTED_EDGE ( 'NONE', *, *, #13218, .F. ) ;
#8274=DIRECTION ( 'NONE',  ( -1.000000000000000000, 0.000000000000000000, 0.000000000000000000 ) ) ;
#8313=ORIENTED_EDGE ( 'NONE', *, *, #31545, .F. ) ;
#8404=DIRECTION ( 'NONE',  ( 0.000000000000000000, -1.000000000000000000, 0.000000000000000000 ) ) ;
#8414=DIRECTION ( 'NONE',  ( -1.000000000000000000, -1.734723475976807094E-16, 0.000000000000000000 ) ) ;
#8421=CARTESIAN_POINT ( 'NONE',  ( -49.99999999999999289, -26.99999999999999645, 113.9999999999999858 ) ) ;
#8429=VECTOR ( 'NONE', #4545, 1000.000000000000000 ) ;
#8437=DIRECTION ( 'NONE',  ( 0.000000000000000000, 0.000000000000000000, 1.000000000000000000 ) ) ;
#8461=ORIENTED_EDGE ( 'NONE', *, *, #16484, .F. ) ;
#8467=ORIENTED_EDGE ( 'NONE', *, *, #269, .T. ) ;
#8476=EDGE_CURVE ( 'NONE', #10703, #14470, #23452, .T. ) ;
#8488=EDGE_LOOP ( 'NONE', ( #22300, #14641, #7734, #30352 ) ) ;
#8495=AXIS2_PLACEMENT_3D ( 'NONE', #2509, #8414, #30396 ) ;
#8500=DIRECTION ( 'NONE',  ( 0.000000000000000000, 0.000000000000000000, 1.000000000000000000 ) ) ;
#8520=DIRECTION ( 'NONE',  ( 0.000000000000000000, -1.000000000000000000, 0.000000000000000000 ) ) ;
#8521=AXIS2_PLACEMENT_3D ( 'NONE', #31086, #28213, #8404 ) ;
#8526=ORIENTED_EDGE ( 'NONE', *, *, #546, .T. ) ;
#8531=ORIENTED_EDGE ( 'NONE', *, *, #20685, .T. ) ;
#8537=CIRCLE ( 'NONE', #497, 6.000000000000002665 ) ;
#8543=DIRECTION ( 'NONE',  ( 1.000000000000000000, 0.000000000000000000, -0.000000000000000000 ) ) ;
#8555=DIRECTION ( 'NONE',  ( 1.000000000000000000, 0.000000000000000000, -0.000000000000000000 ) ) ;
#8572=ORIENTED_EDGE ( 'NONE', *, *, #31314, .T. ) ;
#8582=ORIENTED_EDGE ( 'NONE', *, *, #14899, .T. ) ;
#8583=EDGE_CURVE ( 'NONE', #33867, #30988, #956, .T. ) ;
#8584=VECTOR ( 'NONE', #10609, 1000.000000000000000 ) ;
#8594=EDGE_CURVE ( 'NONE', #33466, #8628, #2708, .T. ) ;
#8597=FACE_OUTER_BOUND ( 'NONE', #31992, .T. ) ;
#8628=VERTEX_POINT ( 'NONE', #16347 ) ;
#8668=AXIS2_PLACEMENT_3D ( 'NONE', #10999, #16903, #28267 ) ;
#8689=CYLINDRICAL_SURFACE ( 'NONE', #18221, 8.000000000000014211 ) ;
#8704=DIRECTION ( 'NONE',  ( 1.734723475976807094E-16, -1.000000000000000000, 0.000000000000000000 ) ) ;
#8729=CARTESIAN_POINT ( 'NONE',  ( 55.00000000000000000, 20.00000000000001776, 120.0000000000000000 ) ) ;
#8748=CARTESIAN_POINT ( 'NONE',  ( 50.00000000000000000, 20.00000000000001776, -15.00000000000001421 ) ) ;
#8763=DIRECTION ( 'NONE',  ( 1.000000000000000000, -0.000000000000000000, -0.000000000000000000 ) ) ;
#8766=CYLINDRICAL_SURFACE ( 'NONE', #10920, 8.000000000000000000 ) ;
#8774=DIRECTION ( 'NONE',  ( -1.000000000000000000, -1.734723475976807094E-16, 0.000000000000000000 ) ) ;
#8842=EDGE_LOOP ( 'NONE', ( #16318, #22400, #16945, #8526, #8582, #10420 ) ) ;
#8866=DIRECTION ( 'NONE',  ( 1.000000000000000000, -0.000000000000000000, -0.000000000000000000 ) ) ;
#8881=LINE ( 'NONE', #33914, #9213 ) ;
#8898=ORIENTED_EDGE ( 'NONE', *, *, #11982, .F. ) ;
#8961=CIRCLE ( 'NONE', #18738, 5.000000000000011546 ) ;
#8964=EDGE_LOOP ( 'NONE', ( #26255, #29726 ) ) ;
#8977=AXIS2_PLACEMENT_3D ( 'NONE', #28169, #33384, #33041 ) ;
#8997=EDGE_CURVE ( 'NONE', #4202, #33867, #20638, .T. ) ;
#9000=DIRECTION ( 'NONE',  ( -1.000000000000000000, 0.000000000000000000, 0.000000000000000000 ) ) ;
#9011=ORIENTED_EDGE ( 'NONE', *, *, #13734, .T. ) ;
#9017=EDGE_LOOP ( 'NONE', ( #5341, #22353 ) ) ;
#9024=ORIENTED_EDGE ( 'NONE', *, *, #10650, .T. ) ;
#9027=AXIS2_PLACEMENT_3D ( 'NONE', #29275, #20779, #29630 ) ;
#9042=CARTESIAN_POINT ( 'NONE',  ( -29.99999999999999645, -26.00000000000000000, 113.9999999999999858 ) ) ;
#9059=AXIS2_PLACEMENT_3D ( 'NONE', #30779, #2739, #25216 ) ;
#9060=FACE_OUTER_BOUND ( 'NONE', #24648, .T. ) ;
#9078=VERTEX_POINT ( 'NONE', #16127 ) ;
#9080=AXIS2_PLACEMENT_3D ( 'NONE', #13322, #21569, #16166 ) ;
#9110=CARTESIAN_POINT ( 'NONE',  ( 55.00000000000000000, 20.00000000000001776, -15.00000000000001421 ) ) ;
#9118=LINE ( 'NONE', #8748, #10774 ) ;
#9160=ORIENTED_EDGE ( 'NONE', *, *, #18073, .T. ) ;
#9177=CIRCLE ( 'NONE', #13212, 11.00000000000000000 ) ;
#9213=VECTOR ( 'NONE', #3864, 1000.000000000000000 ) ;
#9248=CARTESIAN_POINT ( 'NONE',  ( 55.00000000000000000, 6.123233995736780087E-16, 5.000000000000011546 ) ) ;
#9255=FACE_OUTER_BOUND ( 'NONE', #27517, .T. ) ;
#9267=AXIS2_PLACEMENT_3D ( 'NONE', #1080, #25924, #6643 ) ;
#9273=DIRECTION ( 'NONE',  ( 0.000000000000000000, 0.000000000000000000, 1.000000000000000000 ) ) ;
#9283=DIRECTION ( 'NONE',  ( 1.000000000000000000, -0.000000000000000000, -0.000000000000000000 ) ) ;
#9331=DIRECTION ( 'NONE',  ( 0.000000000000000000, 0.000000000000000000, -1.000000000000000000 ) ) ;
#9340=CARTESIAN_POINT ( 'NONE',  ( -50.00000000000000000, -25.98076211353320275, 84.99999999999992895 ) ) ;
#9359=CIRCLE ( 'NONE', #3060, 11.00000000000001066 ) ;
#9380=CYLINDRICAL_SURFACE ( 'NONE', #11577, 7.999999999999992895 ) ;
#9381=CARTESIAN_POINT ( 'NONE',  ( 55.00000000000000000, 20.00000000000001776, 120.0000000000000000 ) ) ;
#9384=CARTESIAN_POINT ( 'NONE',  ( -55.00000000000000000, 10.00000000000000888, -25.00000000000000000 ) ) ;
#9414=EDGE_LOOP ( 'NONE', ( #10581, #5124 ) ) ;
#9416=AXIS2_PLACEMENT_3D ( 'NONE', #10776, #11128, #30214 ) ;
#9438=EDGE_CURVE ( 'NONE', #35006, #28580, #25745, .T. ) ;
#9449=EDGE_CURVE ( 'NONE', #3877, #26571, #10705, .T. ) ;
#9476=CYLINDRICAL_SURFACE ( 'NONE', #32686, 9.999999999999994671 ) ;
#9478=CYLINDRICAL_SURFACE ( 'NONE', #27533, 8.000000000000007105 ) ;
#9527=FACE_OUTER_BOUND ( 'NONE', #24949, .T. ) ;
#9554=EDGE_LOOP ( 'NONE', ( #17339, #25796, #13268, #18185 ) ) ;
#9563=ORIENTED_EDGE ( 'NONE', *, *, #32780, .F. ) ;
#9567=AXIS2_PLACEMENT_3D ( 'NONE', #12438, #32723, #8050 ) ;
#9573=AXIS2_PLACEMENT_3D ( 'NONE', #6055, #13459, #24440 ) ;
#9575=DIRECTION ( 'NONE',  ( 0.000000000000000000, -1.000000000000000000, 0.000000000000000000 ) ) ;
#9594=CARTESIAN_POINT ( 'NONE',  ( -46.00000000000000000, 9.797174393178839462E-16, 61.99999999999999289 ) ) ;
#9624=AXIS2_PLACEMENT_3D ( 'NONE', #15583, #7499, #8035 ) ;
#9641=DIRECTION ( 'NONE',  ( -1.000000000000000000, -1.734723475976807094E-16, 0.000000000000000000 ) ) ;
#9645=DIRECTION ( 'NONE',  ( 0.000000000000000000, -1.000000000000000000, 0.000000000000000000 ) ) ;
#9687=CARTESIAN_POINT ( 'NONE',  ( -55.00000000000000000, -2.775557561562891351E-14, 110.0000000000000000 ) ) ;
#9698=AXIS2_PLACEMENT_3D ( 'NONE', #7840, #2831, #8022 ) ;
#9729=ORIENTED_EDGE ( 'NONE', *, *, #34263, .T. ) ;
#9744=FACE_BOUND ( 'NONE', #25341, .T. ) ;
#9755=AXIS2_PLACEMENT_3D ( 'NONE', #5904, #10963, #17224 ) ;
#9784=CARTESIAN_POINT ( 'NONE',  ( 50.00000000000000000, -59.99999999999997158, 120.0000000000000000 ) ) ;
#9789=ORIENTED_EDGE ( 'NONE', *, *, #29115, .F. ) ;
#9841=EDGE_LOOP ( 'NONE', ( #12343, #11070 ) ) ;
#9866=LINE ( 'NONE', #10241, #33231 ) ;
#9871=ORIENTED_EDGE ( 'NONE', *, *, #33422, .F. ) ;
#9879=ORIENTED_EDGE ( 'NONE', *, *, #29138, .T. ) ;
#9943=VECTOR ( 'NONE', #12875, 1000.000000000000000 ) ;
#9951=CARTESIAN_POINT ( 'NONE',  ( 46.00000000000000000, -25.98076211353320275, 92.99999999999991473 ) ) ;
#9957=CARTESIAN_POINT ( 'NONE',  ( 46.00000000000000000, 1.347111479062090574E-15, 81.00000000000001421 ) ) ;
#9961=DIRECTION ( 'NONE',  ( -0.000000000000000000, -0.000000000000000000, -1.000000000000000000 ) ) ;
#9971=ORIENTED_EDGE ( 'NONE', *, *, #7741, .T. ) ;
#9974=CIRCLE ( 'NONE', #28943, 4.000000000000003553 ) ;
#9976=EDGE_CURVE ( 'NONE', #26571, #28899, #7595, .T. ) ;
#10005=ORIENTED_EDGE ( 'NONE', *, *, #11253, .F. ) ;
#10045=ORIENTED_EDGE ( 'NONE', *, *, #16927, .T. ) ;
#10047=CARTESIAN_POINT ( 'NONE',  ( 55.00000000000000000, -25.98076211353320275, 84.99999999999994316 ) ) ;
#10053=CARTESIAN_POINT ( 'NONE',  ( 46.00000000000000000, 0.000000000000000000, 70.00000000000000000 ) ) ;
#10060=ORIENTED_EDGE ( 'NONE', *, *, #6659, .T. ) ;
#10062=AXIS2_PLACEMENT_3D ( 'NONE', #22094, #5551, #27524 ) ;
#10067=CYLINDRICAL_SURFACE ( 'NONE', #7458, 6.000000000000005329 ) ;
#10097=DIRECTION ( 'NONE',  ( 1.000000000000000000, -0.000000000000000000, -0.000000000000000000 ) ) ;
#10112=ORIENTED_EDGE ( 'NONE', *, *, #20685, .F. ) ;
#10151=ORIENTED_EDGE ( 'NONE', *, *, #34154, .F. ) ;
#10186=MANIFOLD_SOLID_BREP ( 'Mirror1', #19244 ) ;
#10193=AXIS2_PLACEMENT_3D ( 'NONE', #28320, #414, #8520 ) ;
#10198=EDGE_LOOP ( 'NONE', ( #3655, #8531 ) ) ;
#10206=EDGE_CURVE ( 'NONE', #19029, #17795, #1595, .T. ) ;
#10216=AXIS2_PLACEMENT_3D ( 'NONE', #35379, #24752, #33205 ) ;
#10241=CARTESIAN_POINT ( 'NONE',  ( -55.00000000000000000, -25.98076211353320275, 78.99999999999992895 ) ) ;
#10277=EDGE_LOOP ( 'NONE', ( #33558, #26667 ) ) ;
#10288=AXIS2_PLACEMENT_3D ( 'NONE', #19958, #6298, #17266 ) ;
#10301=CARTESIAN_POINT ( 'NONE',  ( -46.00000000000000000, -25.98076211353320275, 84.99999999999992895 ) ) ;
#10380=ADVANCED_FACE ( 'NONE', ( #17372 ), #13979, .F. ) ;
#10402=ADVANCED_FACE ( 'NONE', ( #28557 ), #14321, .T. ) ;
#10420=ORIENTED_EDGE ( 'NONE', *, *, #24504, .T. ) ;
#10422=CARTESIAN_POINT ( 'NONE',  ( -46.00000000000000000, -25.98076211353320275, 95.99999999999991473 ) ) ;
#10436=ORIENTED_EDGE ( 'NONE', *, *, #33892, .F. ) ;
#10437=CARTESIAN_POINT ( 'NONE',  ( -46.00000000000000000, 1.347111479062090180E-15, 59.00000000000000000 ) ) ;
#10442=DIRECTION ( 'NONE',  ( 1.000000000000000000, -0.000000000000000000, -0.000000000000000000 ) ) ;
#10486=CARTESIAN_POINT ( 'NONE',  ( 54.99999999999999289, -64.99999999999997158, 120.0000000000000000 ) ) ;
#10487=ORIENTED_EDGE ( 'NONE', *, *, #15461, .T. ) ;
#10540=AXIS2_PLACEMENT_3D ( 'NONE', #676, #8774, #19741 ) ;
#10570=EDGE_CURVE ( 'NONE', #9078, #26450, #34859, .T. ) ;
#10581=ORIENTED_EDGE ( 'NONE', *, *, #34263, .F. ) ;
#10584=DIRECTION ( 'NONE',  ( 0.000000000000000000, 0.000000000000000000, -1.000000000000000000 ) ) ;
#10595=EDGE_CURVE ( 'NONE', #26801, #32964, #13253, .T. ) ;
#10609=DIRECTION ( 'NONE',  ( -1.000000000000000000, -0.000000000000000000, -0.000000000000000000 ) ) ;
#10623=ORIENTED_EDGE ( 'NONE', *, *, #17892, .F. ) ;
#10647=EDGE_LOOP ( 'NONE', ( #7972, #12904, #1069, #22324 ) ) ;
#10650=EDGE_CURVE ( 'NONE', #24282, #35000, #18272, .T. ) ;
#10703=VERTEX_POINT ( 'NONE', #30158 ) ;
#10705=LINE ( 'NONE', #21675, #33189 ) ;
#10711=VERTEX_POINT ( 'NONE', #16453 ) ;
#10729=PRESENTATION_STYLE_ASSIGNMENT (( #7657 ) ) ;
#10738=ORIENTED_EDGE ( 'NONE', *, *, #34015, .F. ) ;
#10743=VECTOR ( 'NONE', #9283, 1000.000000000000000 ) ;
#10774=VECTOR ( 'NONE', #14680, 1000.000000000000000 ) ;
#10776=CARTESIAN_POINT ( 'NONE',  ( 50.00000000000000711, -2.775557561562891351E-14, 110.0000000000000000 ) ) ;
#10780=CARTESIAN_POINT ( 'NONE',  ( -55.00000000000000000, 0.000000000000000000, 70.00000000000000000 ) ) ;
#10790=VECTOR ( 'NONE', #24502, 1000.000000000000000 ) ;
#10812=ORIENTED_EDGE ( 'NONE', *, *, #3429, .T. ) ;
#10848=EDGE_CURVE ( 'NONE', #864, #32025, #8881, .T. ) ;
#10849=VERTEX_POINT ( 'NONE', #9248 ) ;
#10853=CARTESIAN_POINT ( 'NONE',  ( -46.00000000000000000, 0.000000000000000000, 11.00000000000000000 ) ) ;
#10858=DIRECTION ( 'NONE',  ( 1.000000000000000000, -0.000000000000000000, -0.000000000000000000 ) ) ;
#10913=EDGE_LOOP ( 'NONE', ( #33706, #23319, #6990, #8227, #4017, #8572, #5390, #15432 ) ) ;
#10919=ORIENTED_EDGE ( 'NONE', *, *, #34176, .T. ) ;
#10920=AXIS2_PLACEMENT_3D ( 'NONE', #3042, #19734, #11314 ) ;
#10925=FACE_BOUND ( 'NONE', #9017, .T. ) ;
#10939=CIRCLE ( 'NONE', #31052, 6.000000000000005329 ) ;
#10949=VERTEX_POINT ( 'NONE', #14283 ) ;
#10959=CARTESIAN_POINT ( 'NONE',  ( 50.00000000000000711, -25.98076211353320275, 84.99999999999994316 ) ) ;
#10963=DIRECTION ( 'NONE',  ( -1.000000000000000000, -1.734723475976807094E-16, 0.000000000000000000 ) ) ;
#10964=VECTOR ( 'NONE', #15771, 1000.000000000000000 ) ;
#10999=CARTESIAN_POINT ( 'NONE',  ( 46.00000000000000000, 0.000000000000000000, 0.000000000000000000 ) ) ;
#11010=LINE ( 'NONE', #13881, #29249 ) ;
#11054=EDGE_CURVE ( 'NONE', #22703, #32586, #26354, .T. ) ;
#11070=ORIENTED_EDGE ( 'NONE', *, *, #33422, .T. ) ;
#11072=DIRECTION ( 'NONE',  ( -0.000000000000000000, 0.000000000000000000, 1.000000000000000000 ) ) ;
#11084=ORIENTED_EDGE ( 'NONE', *, *, #7098, .T. ) ;
#11088=AXIS2_PLACEMENT_3D ( 'NONE', #20671, #31667, #26463 ) ;
#11089=VERTEX_POINT ( 'NONE', #20918 ) ;
#11090=ORIENTED_EDGE ( 'NONE', *, *, #28887, .T. ) ;
#11128=DIRECTION ( 'NONE',  ( 1.000000000000000000, 0.000000000000000000, -0.000000000000000000 ) ) ;
#11158=VERTEX_POINT ( 'NONE', #26538 ) ;
#11163=CARTESIAN_POINT ( 'NONE',  ( 46.00000000000000000, 0.000000000000000000, 0.000000000000000000 ) ) ;
#11168=VERTEX_POINT ( 'NONE', #9957 ) ;
#11169=ORIENTED_EDGE ( 'NONE', *, *, #18934, .T. ) ;
#11215=CIRCLE ( 'NONE', #5494, 6.000000000000005329 ) ;
#11216=EDGE_CURVE ( 'NONE', #7646, #3309, #20138, .T. ) ;
#11217=PRODUCT_DEFINITION_CONTEXT ( 'detailed design', #18159, 'design' ) ;
#11221=ADVANCED_FACE ( 'NONE', ( #2587 ), #30297, .T. ) ;
#11230=PLANE ( 'NONE',  #34162 ) ;
#11253=EDGE_CURVE ( 'NONE', #30036, #17467, #28802, .T. ) ;
#11258=FACE_OUTER_BOUND ( 'NONE', #16587, .T. ) ;
#11271=AXIS2_PLACEMENT_3D ( 'NONE', #1730, #25874, #31258 ) ;
#11276=ADVANCED_FACE ( 'NONE', ( #35531 ), #2410, .T. ) ;
#11280=DIRECTION ( 'NONE',  ( 0.000000000000000000, 0.000000000000000000, -1.000000000000000000 ) ) ;
#11297=EDGE_CURVE ( 'NONE', #15120, #32416, #2773, .T. ) ;
#11314=DIRECTION ( 'NONE',  ( 0.000000000000000000, 0.000000000000000000, -1.000000000000000000 ) ) ;
#11331=ORIENTED_EDGE ( 'NONE', *, *, #11216, .T. ) ;
#11360=CIRCLE ( 'NONE', #14790, 6.000000000000005329 ) ;
#11375=AXIS2_PLACEMENT_3D ( 'NONE', #22502, #195, #28277 ) ;
#11388=AXIS2_PLACEMENT_3D ( 'NONE', #10047, #12936, #32198 ) ;
#11405=CARTESIAN_POINT ( 'NONE',  ( 50.00000000000000000, 0.000000000000000000, 0.000000000000000000 ) ) ;
#11412=ADVANCED_FACE ( 'NONE', ( #564 ), #9380, .F. ) ;
#11418=CARTESIAN_POINT ( 'NONE',  ( -50.00000000000000000, -25.98076211353320275, 95.99999999999991473 ) ) ;
#11449=LINE ( 'NONE', #19365, #29531 ) ;
#11457=ORIENTED_EDGE ( 'NONE', *, *, #20666, .T. ) ;
#11486=FACE_BOUND ( 'NONE', #21989, .T. ) ;
#11569=FACE_OUTER_BOUND ( 'NONE', #31737, .T. ) ;
#11577=AXIS2_PLACEMENT_3D ( 'NONE', #27774, #28471, #16932 ) ;
#11595=CARTESIAN_POINT ( 'NONE',  ( -46.00000000000000000, 0.000000000000000000, 70.00000000000000000 ) ) ;
#11600=CIRCLE ( 'NONE', #15591, 7.999999999999992895 ) ;
#11610=EDGE_CURVE ( 'NONE', #16063, #30657, #17315, .T. ) ;
#11670=ORIENTED_EDGE ( 'NONE', *, *, #11297, .F. ) ;
#11681=AXIS2_PLACEMENT_3D ( 'NONE', #32740, #5560, #7709 ) ;
#11697=VERTEX_POINT ( 'NONE', #25534 ) ;
#11736=EDGE_LOOP ( 'NONE', ( #11331, #8088 ) ) ;
#11739=EDGE_LOOP ( 'NONE', ( #20687, #12972, #14300, #25652 ) ) ;
#11750=UNCERTAINTY_MEASURE_WITH_UNIT (LENGTH_MEASURE( 1.000000000000000082E-05 ), #27484, 'distance_accuracy_value', 'NONE');
#11761=FACE_OUTER_BOUND ( 'NONE', #8065, .T. ) ;
#11796=LINE ( 'NONE', #33582, #10743 ) ;
#11817=AXIS2_PLACEMENT_3D ( 'NONE', #253, #16974, #30155 ) ;
#11825=LINE ( 'NONE', #12366, #15615 ) ;
#11855=CIRCLE ( 'NONE', #29709, 6.000000000000005329 ) ;
#11880=CIRCLE ( 'NONE', #3267, 10.00000000000000000 ) ;
#11884=FACE_OUTER_BOUND ( 'NONE', #8488, .T. ) ;
#11889=CARTESIAN_POINT ( 'NONE',  ( 46.00000000000000000, 0.000000000000000000, 59.00000000000000000 ) ) ;
#11907=EDGE_LOOP ( 'NONE', ( #14917, #25876, #20658, #31863 ) ) ;
#11941=AXIS2_PLACEMENT_3D ( 'NONE', #18913, #31885, #32075 ) ;
#11947=CIRCLE ( 'NONE', #2188, 8.000000000000007105 ) ;
#11964=ORIENTED_EDGE ( 'NONE', *, *, #8583, .T. ) ;
#11982=EDGE_CURVE ( 'NONE', #6343, #16796, #33442, .T. ) ;
#12003=DIRECTION ( 'NONE',  ( 0.000000000000000000, 0.000000000000000000, 1.000000000000000000 ) ) ;
#12005=ORIENTED_EDGE ( 'NONE', *, *, #23577, .F. ) ;
#12008=DIRECTION ( 'NONE',  ( 1.000000000000000000, -0.000000000000000000, 0.000000000000000000 ) ) ;
#12018=VERTEX_POINT ( 'NONE', #27397 ) ;
#12042=ORIENTED_EDGE ( 'NONE', *, *, #2000, .F. ) ;
#12087=ADVANCED_BREP_SHAPE_REPRESENTATION ( '', ( #10186, #21307 ), #13295 ) ;
#12121=CARTESIAN_POINT ( 'NONE',  ( -55.00000000000000000, -25.98076211353320275, 84.99999999999994316 ) ) ;
#12131=CYLINDRICAL_SURFACE ( 'NONE', #33708, 10.99999999999999645 ) ;
#12151=DIRECTION ( 'NONE',  ( 1.000000000000000000, 0.000000000000000000, 0.000000000000000000 ) ) ;
#12162=DIRECTION ( 'NONE',  ( -1.000000000000000000, -0.000000000000000000, -0.000000000000000000 ) ) ;
#12177=EDGE_CURVE ( 'NONE', #10949, #17665, #11825, .T. ) ;
#12181=ORIENTED_EDGE ( 'NONE', *, *, #10570, .T. ) ;
#12187=CARTESIAN_POINT ( 'NONE',  ( -46.00000000000000000, 9.797174393178825657E-16, -8.000000000000000000 ) ) ;
#12222=CARTESIAN_POINT ( 'NONE',  ( 50.00000000000000000, 1.347111479062088405E-15, 11.00000000000000000 ) ) ;
#12230=FACE_OUTER_BOUND ( 'NONE', #16013, .T. ) ;
#12300=EDGE_CURVE ( 'NONE', #11168, #22745, #17936, .T. ) ;
#12310=CARTESIAN_POINT ( 'NONE',  ( 46.00000000000000000, 0.000000000000000000, -11.00000000000000000 ) ) ;
#12335=FACE_BOUND ( 'NONE', #12894, .T. ) ;
#12343=ORIENTED_EDGE ( 'NONE', *, *, #14474, .T. ) ;
#12353=ORIENTED_EDGE ( 'NONE', *, *, #17822, .F. ) ;
#12366=CARTESIAN_POINT ( 'NONE',  ( 46.00000000000000000, 9.797174393178825657E-16, 8.000000000000000000 ) ) ;
#12401=ORIENTED_EDGE ( 'NONE', *, *, #17864, .T. ) ;
#12413=ORIENTED_EDGE ( 'NONE', *, *, #4280, .F. ) ;
#12438=CARTESIAN_POINT ( 'NONE',  ( 46.00000000000000000, -25.98076211353320275, 84.99999999999992895 ) ) ;
#12462=ORIENTED_EDGE ( 'NONE', *, *, #16722, .F. ) ;
#12489=LINE ( 'NONE', #9784, #17630 ) ;
#12498=ORIENTED_EDGE ( 'NONE', *, *, #32968, .F. ) ;
#12503=VECTOR ( 'NONE', #15410, 1000.000000000000000 ) ;
#12529=ORIENTED_EDGE ( 'NONE', *, *, #34154, .T. ) ;
#12547=DIRECTION ( 'NONE',  ( -1.000000000000000000, -0.000000000000000000, -0.000000000000000000 ) ) ;
#12565=ADVANCED_FACE ( 'NONE', ( #30363, #279 ), #33573, .F. ) ;
#12573=CYLINDRICAL_SURFACE ( 'NONE', #2119, 0.9999999999999974465 ) ;
#12627=DIRECTION ( 'NONE',  ( 0.000000000000000000, 0.000000000000000000, -1.000000000000000000 ) ) ;
#12642=ORIENTED_EDGE ( 'NONE', *, *, #10848, .T. ) ;
#12660=DIRECTION ( 'NONE',  ( -0.000000000000000000, -0.000000000000000000, -1.000000000000000000 ) ) ;
#12666=ORIENTED_EDGE ( 'NONE', *, *, #11297, .T. ) ;
#12703=LINE ( 'NONE', #7290, #13049 ) ;
#12711=AXIS2_PLACEMENT_3D ( 'NONE', #26783, #23351, #7146 ) ;
#12724=AXIS2_PLACEMENT_3D ( 'NONE', #10780, #21742, #5555 ) ;
#12725=DIRECTION ( 'NONE',  ( 0.000000000000000000, 0.000000000000000000, 1.000000000000000000 ) ) ;
#12761=EDGE_CURVE ( 'NONE', #28899, #19518, #24158, .T. ) ;
#12764=DIRECTION ( 'NONE',  ( 0.000000000000000000, 0.000000000000000000, -1.000000000000000000 ) ) ;
#12802=CARTESIAN_POINT ( 'NONE',  ( -55.00000000000000000, 0.000000000000000000, 0.000000000000000000 ) ) ;
#12804=EDGE_CURVE ( 'NONE', #30169, #34014, #23000, .T. ) ;
#12807=DIRECTION ( 'NONE',  ( -0.000000000000000000, -0.000000000000000000, -1.000000000000000000 ) ) ;
#12812=FACE_OUTER_BOUND ( 'NONE', #3102, .T. ) ;
#12815=ORIENTED_EDGE ( 'NONE', *, *, #32745, .T. ) ;
#12818=CARTESIAN_POINT ( 'NONE',  ( -49.99999999999999289, -26.99999999999999645, 113.9999999999999858 ) ) ;
#12819=EDGE_LOOP ( 'NONE', ( #31866, #33088, #29829, #9563 ) ) ;
#12825=VERTEX_POINT ( 'NONE', #330 ) ;
#12852=CARTESIAN_POINT ( 'NONE',  ( 55.00000000000000000, 20.00000000000001776, 120.0000000000000000 ) ) ;
#12875=DIRECTION ( 'NONE',  ( -1.000000000000000000, -1.387778780781445922E-16, 0.000000000000000000 ) ) ;
#12886=DIRECTION ( 'NONE',  ( 1.000000000000000000, -0.000000000000000000, -0.000000000000000000 ) ) ;
#12887=DIRECTION ( 'NONE',  ( -1.000000000000000000, -0.000000000000000000, -0.000000000000000000 ) ) ;
#12894=EDGE_LOOP ( 'NONE', ( #10060, #18854 ) ) ;
#12897=DIRECTION ( 'NONE',  ( 0.000000000000000000, 0.000000000000000000, 1.000000000000000000 ) ) ;
#12904=ORIENTED_EDGE ( 'NONE', *, *, #7098, .F. ) ;
#12913=DIRECTION ( 'NONE',  ( 0.000000000000000000, 0.000000000000000000, 1.000000000000000000 ) ) ;
#12936=DIRECTION ( 'NONE',  ( 1.000000000000000000, 0.000000000000000000, 0.000000000000000000 ) ) ;
#12969=CARTESIAN_POINT ( 'NONE',  ( -55.00000000000000000, 10.00000000000000888, 120.0000000000000000 ) ) ;
#12972=ORIENTED_EDGE ( 'NONE', *, *, #7699, .T. ) ;
#12978=AXIS2_PLACEMENT_3D ( 'NONE', #26212, #26758, #29632 ) ;
#13047=EDGE_CURVE ( 'NONE', #33645, #2204, #28949, .T. ) ;
#13049=VECTOR ( 'NONE', #18264, 1000.000000000000000 ) ;
#13087=ORIENTED_EDGE ( 'NONE', *, *, #29115, .T. ) ;
#13095=CIRCLE ( 'NONE', #9059, 8.000000000000007105 ) ;
#13136=DIRECTION ( 'NONE',  ( 1.000000000000000000, 1.734723475976807094E-16, 0.000000000000000000 ) ) ;
#13145=CARTESIAN_POINT ( 'NONE',  ( 54.99999999999999289, -64.99999999999997158, 120.0000000000000000 ) ) ;
#13146=CARTESIAN_POINT ( 'NONE',  ( -54.99999999999998579, -64.99999999999997158, -25.00000000000000000 ) ) ;
#13149=CARTESIAN_POINT ( 'NONE',  ( 55.00000000000000000, -25.98076211353320275, 90.99999999999994316 ) ) ;
#13194=CARTESIAN_POINT ( 'NONE',  ( -46.00000000000000000, 9.797174393178825657E-16, -8.000000000000000000 ) ) ;
#13212=AXIS2_PLACEMENT_3D ( 'NONE', #13836, #505, #32925 ) ;
#13218=EDGE_CURVE ( 'NONE', #2874, #19260, #25337, .T. ) ;
#13225=ORIENTED_EDGE ( 'NONE', *, *, #16234, .T. ) ;
#13247=DIRECTION ( 'NONE',  ( 1.000000000000000000, -0.000000000000000000, -0.000000000000000000 ) ) ;
#13253=LINE ( 'NONE', #2099, #15519 ) ;
#13268=ORIENTED_EDGE ( 'NONE', *, *, #17822, .T. ) ;
#13271=CYLINDRICAL_SURFACE ( 'NONE', #9698, 6.000000000000005329 ) ;
#13295=( GEOMETRIC_REPRESENTATION_CONTEXT ( 3 ) GLOBAL_UNCERTAINTY_ASSIGNED_CONTEXT ( ( #11750 ) ) GLOBAL_UNIT_ASSIGNED_CONTEXT ( ( #27484, #33052, #15936 ) ) REPRESENTATION_CONTEXT ( 'NONE', 'WORKASPACE' ) );
#13306=ORIENTED_EDGE ( 'NONE', *, *, #19602, .T. ) ;
#13322=CARTESIAN_POINT ( 'NONE',  ( -49.99999999999999289, -25.98076211353320275, 84.99999999999994316 ) ) ;
#13352=DIRECTION ( 'NONE',  ( 1.000000000000000000, -0.000000000000000000, -0.000000000000000000 ) ) ;
#13366=DIRECTION ( 'NONE',  ( 1.000000000000000000, 0.000000000000000000, 0.000000000000000000 ) ) ;
#13367=CARTESIAN_POINT ( 'NONE',  ( -55.00000000000000000, 0.000000000000000000, 70.00000000000000000 ) ) ;
#13387=VERTEX_POINT ( 'NONE', #470 ) ;
#13407=EDGE_CURVE ( 'NONE', #21242, #14544, #11796, .T. ) ;
#13427=EDGE_CURVE ( 'NONE', #17487, #28349, #33777, .T. ) ;
#13439=EDGE_CURVE ( 'NONE', #11158, #28784, #11880, .T. ) ;
#13459=DIRECTION ( 'NONE',  ( -1.000000000000000000, -1.734723475976807094E-16, 0.000000000000000000 ) ) ;
#13469=ORIENTED_EDGE ( 'NONE', *, *, #2260, .T. ) ;
#13477=EDGE_CURVE ( 'NONE', #31888, #35006, #1013, .T. ) ;
#13478=FACE_OUTER_BOUND ( 'NONE', #32425, .T. ) ;
#13480=ORIENTED_EDGE ( 'NONE', *, *, #546, .F. ) ;
#13485=DIRECTION ( 'NONE',  ( 0.000000000000000000, 0.000000000000000000, -1.000000000000000000 ) ) ;
#13504=EDGE_LOOP ( 'NONE', ( #27020, #23191 ) ) ;
#13508=FACE_BOUND ( 'NONE', #20448, .T. ) ;
#13520=CARTESIAN_POINT ( 'NONE',  ( 0.000000000000000000, 10.00000000000000888, -25.00000000000000000 ) ) ;
#13543=EDGE_LOOP ( 'NONE', ( #3324, #12529, #24691, #7639 ) ) ;
#13551=DIRECTION ( 'NONE',  ( 0.000000000000000000, 0.000000000000000000, -1.000000000000000000 ) ) ;
#13594=CARTESIAN_POINT ( 'NONE',  ( -55.00000000000000000, 0.000000000000000000, -5.000000000000011546 ) ) ;
#13617=ADVANCED_FACE ( 'NONE', ( #12335, #6936 ), #29086, .F. ) ;
#13618=FACE_OUTER_BOUND ( 'NONE', #10277, .T. ) ;
#13637=DIRECTION ( 'NONE',  ( -1.734723475976807094E-16, 1.000000000000000000, 0.000000000000000000 ) ) ;
#13724=AXIS2_PLACEMENT_3D ( 'NONE', #28139, #22361, #33357 ) ;
#13734=EDGE_CURVE ( 'NONE', #14470, #10711, #2811, .T. ) ;
#13736=CARTESIAN_POINT ( 'NONE',  ( -55.00000000000000000, 0.000000000000000000, 64.00000000000000000 ) ) ;
#13740=ORIENTED_EDGE ( 'NONE', *, *, #32968, .T. ) ;
#13753=LINE ( 'NONE', #20798, #17714 ) ;
#13769=CARTESIAN_POINT ( 'NONE',  ( -55.00000000000000000, 0.000000000000000000, -5.000000000000011546 ) ) ;
#13792=ORIENTED_EDGE ( 'NONE', *, *, #16484, .T. ) ;
#13836=CARTESIAN_POINT ( 'NONE',  ( -50.00000000000000000, 0.000000000000000000, 0.000000000000000000 ) ) ;
#13857=FACE_OUTER_BOUND ( 'NONE', #20801, .T. ) ;
#13861=CARTESIAN_POINT ( 'NONE',  ( -50.00000000000000000, 7.347880794884119736E-16, 76.00000000000001421 ) ) ;
#13881=CARTESIAN_POINT ( 'NONE',  ( -55.00000000000000000, 0.000000000000000000, 64.00000000000000000 ) ) ;
#13908=CARTESIAN_POINT ( 'NONE',  ( -50.00000000000000000, 9.797174393178839462E-16, 61.99999999999999289 ) ) ;
#13924=EDGE_CURVE ( 'NONE', #11089, #28349, #7878, .T. ) ;
#13926=CARTESIAN_POINT ( 'NONE',  ( 50.00000000000000000, 10.00000000000000888, 110.0000000000000000 ) ) ;
#13966=FACE_OUTER_BOUND ( 'NONE', #1030, .T. ) ;
#13968=CARTESIAN_POINT ( 'NONE',  ( -46.00000000000000000, -25.98076211353320275, 84.99999999999992895 ) ) ;
#13971=SHAPE_REPRESENTATION ( 'Mounting Base Plate Frame', ( #21307 ), #13295 ) ;
#13972=FACE_BOUND ( 'NONE', #19629, .T. ) ;
#13979=CYLINDRICAL_SURFACE ( 'NONE', #19528, 8.000000000000000000 ) ;
#14014=DIRECTION ( 'NONE',  ( -1.000000000000000000, 0.000000000000000000, 0.000000000000000000 ) ) ;
#14034=CARTESIAN_POINT ( 'NONE',  ( 46.00000000000000000, 0.000000000000000000, 70.00000000000000000 ) ) ;
#14046=CARTESIAN_POINT ( 'NONE',  ( 46.00000000000000000, -25.98076211353320275, 84.99999999999992895 ) ) ;
#14070=DIRECTION ( 'NONE',  ( 0.000000000000000000, 0.000000000000000000, -1.000000000000000000 ) ) ;
#14090=CARTESIAN_POINT ( 'NONE',  ( 46.00000000000000000, 0.000000000000000000, 70.00000000000000000 ) ) ;
#14093=EDGE_CURVE ( 'NONE', #864, #33645, #344, .T. ) ;
#14109=DIRECTION ( 'NONE',  ( 0.000000000000000000, -1.000000000000000000, 0.000000000000000000 ) ) ;
#14140=DIRECTION ( 'NONE',  ( -0.000000000000000000, 0.000000000000000000, -1.000000000000000000 ) ) ;
#14143=CIRCLE ( 'NONE', #19304, 7.999999999999992895 ) ;
#14205=ADVANCED_FACE ( 'NONE', ( #4095 ), #1024, .T. ) ;
#14227=DIRECTION ( 'NONE',  ( 0.000000000000000000, 0.000000000000000000, 1.000000000000000000 ) ) ;
#14235=ORIENTED_EDGE ( 'NONE', *, *, #11054, .F. ) ;
#14239=AXIS2_PLACEMENT_3D ( 'NONE', #34382, #23384, #25747 ) ;
#14253=EDGE_LOOP ( 'NONE', ( #31142, #30121, #14956, #16371 ) ) ;
#14276=CARTESIAN_POINT ( 'NONE',  ( 50.00000000000000000, 10.00000000000000888, -25.00000000000000000 ) ) ;
#14283=CARTESIAN_POINT ( 'NONE',  ( 46.00000000000000000, 9.797174393178825657E-16, 8.000000000000000000 ) ) ;
#14287=CARTESIAN_POINT ( 'NONE',  ( -49.99999999999998579, -64.99999999999997158, 120.0000000000000000 ) ) ;
#14290=CIRCLE ( 'NONE', #16009, 10.99999999999999645 ) ;
#14300=ORIENTED_EDGE ( 'NONE', *, *, #33892, .T. ) ;
#14312=FACE_OUTER_BOUND ( 'NONE', #25297, .T. ) ;
#14321=CYLINDRICAL_SURFACE ( 'NONE', #16654, 10.99999999999999645 ) ;
#14330=ORIENTED_EDGE ( 'NONE', *, *, #17735, .T. ) ;
#14407=ORIENTED_EDGE ( 'NONE', *, *, #35480, .T. ) ;
#14410=DIRECTION ( 'NONE',  ( 0.000000000000000000, 0.000000000000000000, -1.000000000000000000 ) ) ;
#14411=ORIENTED_EDGE ( 'NONE', *, *, #33687, .F. ) ;
#14448=DIRECTION ( 'NONE',  ( 1.000000000000000000, 1.734723475976807094E-16, 0.000000000000000000 ) ) ;
#14470=VERTEX_POINT ( 'NONE', #2454 ) ;
#14474=EDGE_CURVE ( 'NONE', #17673, #19029, #11855, .T. ) ;
#14499=CARTESIAN_POINT ( 'NONE',  ( 50.00000000000000000, -25.98076211353320275, 76.99999999999992895 ) ) ;
#14506=AXIS2_PLACEMENT_3D ( 'NONE', #30620, #17273, #28278 ) ;
#14507=CARTESIAN_POINT ( 'NONE',  ( -55.00000000000000000, 0.000000000000000000, -5.000000000000011546 ) ) ;
#14512=EDGE_CURVE ( 'NONE', #24505, #25823, #21869, .T. ) ;
#14522=VECTOR ( 'NONE', #15953, 1000.000000000000000 ) ;
#14544=VERTEX_POINT ( 'NONE', #438 ) ;
#14554=DIRECTION ( 'NONE',  ( 0.000000000000000000, -1.000000000000000000, 0.000000000000000000 ) ) ;
#14596=PLANE ( 'NONE',  #34920 ) ;
#14598=ORIENTED_EDGE ( 'NONE', *, *, #13924, .T. ) ;
#14611=DIRECTION ( 'NONE',  ( -0.000000000000000000, -0.000000000000000000, -1.000000000000000000 ) ) ;
#14639=CARTESIAN_POINT ( 'NONE',  ( 46.00000000000000000, -25.98076211353320275, 92.99999999999991473 ) ) ;
#14641=ORIENTED_EDGE ( 'NONE', *, *, #13218, .T. ) ;
#14651=AXIS2_PLACEMENT_3D ( 'NONE', #18932, #18753, #7593 ) ;
#14680=DIRECTION ( 'NONE',  ( -1.000000000000000000, 0.000000000000000000, -0.000000000000000000 ) ) ;
#14721=DIRECTION ( 'NONE',  ( 1.000000000000000000, 0.000000000000000000, -0.000000000000000000 ) ) ;
#14735=CYLINDRICAL_SURFACE ( 'NONE', #14239, 5.000000000000011546 ) ;
#14749=AXIS2_PLACEMENT_3D ( 'NONE', #25869, #1193, #9645 ) ;
#14777=LINE ( 'NONE', #9381, #15151 ) ;
#14790=AXIS2_PLACEMENT_3D ( 'NONE', #33221, #8543, #5850 ) ;
#14808=EDGE_CURVE ( 'NONE', #17845, #3877, #12489, .T. ) ;
#14813=CARTESIAN_POINT ( 'NONE',  ( -49.99999999999999289, -26.00000000000000000, 113.9999999999999858 ) ) ;
#14868=DIRECTION ( 'NONE',  ( 0.000000000000000000, 0.000000000000000000, -1.000000000000000000 ) ) ;
#14877=ORIENTED_EDGE ( 'NONE', *, *, #28577, .T. ) ;
#14896=CYLINDRICAL_SURFACE ( 'NONE', #22180, 8.000000000000014211 ) ;
#14899=EDGE_CURVE ( 'NONE', #18111, #23442, #7252, .T. ) ;
#14917=ORIENTED_EDGE ( 'NONE', *, *, #14808, .T. ) ;
#14919=CARTESIAN_POINT ( 'NONE',  ( -55.00000000000000000, 6.123233995736780087E-16, 5.000000000000011546 ) ) ;
#14922=CIRCLE ( 'NONE', #19923, 8.000000000000007105 ) ;
#14943=ORIENTED_EDGE ( 'NONE', *, *, #24591, .T. ) ;
#14956=ORIENTED_EDGE ( 'NONE', *, *, #15129, .T. ) ;
#14982=MECHANICAL_DESIGN_GEOMETRIC_PRESENTATION_REPRESENTATION('',(#30529),#623);
#14998=CYLINDRICAL_SURFACE ( 'NONE', #25442, 7.999999999999992895 ) ;
#15101=DIRECTION ( 'NONE',  ( -1.000000000000000000, -1.734723475976807094E-16, -0.000000000000000000 ) ) ;
#15120=VERTEX_POINT ( 'NONE', #16767 ) ;
#15126=AXIS2_PLACEMENT_3D ( 'NONE', #16836, #35601, #3183 ) ;
#15129=EDGE_CURVE ( 'NONE', #1992, #22338, #21669, .T. ) ;
#15151=VECTOR ( 'NONE', #12807, 1000.000000000000000 ) ;
#15180=EDGE_CURVE ( 'NONE', #33007, #25823, #25702, .T. ) ;
#15199=CARTESIAN_POINT ( 'NONE',  ( -46.00000000000000000, 9.797174393178841435E-16, 61.99999999999999289 ) ) ;
#15211=ADVANCED_FACE ( 'NONE', ( #6867 ), #23067, .F. ) ;
#15245=CARTESIAN_POINT ( 'NONE',  ( 46.00000000000000000, 0.000000000000000000, 70.00000000000000000 ) ) ;
#15257=EDGE_LOOP ( 'NONE', ( #30801, #6068 ) ) ;
#15264=DIRECTION ( 'NONE',  ( 0.000000000000000000, 0.000000000000000000, 1.000000000000000000 ) ) ;
#15272=CARTESIAN_POINT ( 'NONE',  ( 46.00000000000000000, 0.000000000000000000, 0.000000000000000000 ) ) ;
#15281=DIRECTION ( 'NONE',  ( 1.000000000000000000, 0.000000000000000000, -0.000000000000000000 ) ) ;
#15308=VERTEX_POINT ( 'NONE', #25965 ) ;
#15319=EDGE_LOOP ( 'NONE', ( #20526, #1738, #23231, #17440 ) ) ;
#15320=ORIENTED_EDGE ( 'NONE', *, *, #13047, .F. ) ;
#15324=LINE ( 'NONE', #20360, #19097 ) ;
#15331=CIRCLE ( 'NONE', #15930, 11.00000000000000000 ) ;
#15342=CIRCLE ( 'NONE', #35505, 8.000000000000000000 ) ;
#15397=VECTOR ( 'NONE', #3595, 1000.000000000000000 ) ;
#15410=DIRECTION ( 'NONE',  ( 1.000000000000000000, -0.000000000000000000, -0.000000000000000000 ) ) ;
#15413=DIRECTION ( 'NONE',  ( 0.000000000000000000, 0.000000000000000000, 1.000000000000000000 ) ) ;
#15429=CARTESIAN_POINT ( 'NONE',  ( -50.00000000000000000, -25.98076211353320275, 84.99999999999992895 ) ) ;
#15432=ORIENTED_EDGE ( 'NONE', *, *, #21312, .F. ) ;
#15451=LINE ( 'NONE', #26467, #25288 ) ;
#15461=EDGE_CURVE ( 'NONE', #2204, #32025, #27487, .T. ) ;
#15472=VECTOR ( 'NONE', #4491, 1000.000000000000000 ) ;
#15477=DIRECTION ( 'NONE',  ( 1.000000000000000000, -0.000000000000000000, -0.000000000000000000 ) ) ;
#15489=CIRCLE ( 'NONE', #20672, 5.000000000000011546 ) ;
#15519=VECTOR ( 'NONE', #23870, 1000.000000000000000 ) ;
#15564=CARTESIAN_POINT ( 'NONE',  ( -49.99999999999999289, -25.98076211353320275, 84.99999999999992895 ) ) ;
#15581=EDGE_CURVE ( 'NONE', #24282, #16219, #13095, .T. ) ;
#15583=CARTESIAN_POINT ( 'NONE',  ( 55.00000000000000000, -2.775557561562891351E-14, 110.0000000000000000 ) ) ;
#15585=DIRECTION ( 'NONE',  ( 1.000000000000000000, 0.000000000000000000, 0.000000000000000000 ) ) ;
#15591=AXIS2_PLACEMENT_3D ( 'NONE', #22982, #1037, #6255 ) ;
#15597=PRESENTATION_STYLE_ASSIGNMENT (( #24270 ) ) ;
#15610=EDGE_CURVE ( 'NONE', #11168, #4839, #17088, .T. ) ;
#15615=VECTOR ( 'NONE', #20268, 1000.000000000000000 ) ;
#15640=DIRECTION ( 'NONE',  ( 0.000000000000000000, -1.000000000000000000, 0.000000000000000000 ) ) ;
#15663=ORIENTED_EDGE ( 'NONE', *, *, #33847, .F. ) ;
#15668=FACE_OUTER_BOUND ( 'NONE', #35174, .T. ) ;
#15672=CIRCLE ( 'NONE', #5348, 5.000000000000011546 ) ;
#15740=CYLINDRICAL_SURFACE ( 'NONE', #12978, 7.999999999999992895 ) ;
#15751=ORIENTED_EDGE ( 'NONE', *, *, #23395, .T. ) ;
#15761=CARTESIAN_POINT ( 'NONE',  ( -55.00000000000000000, -2.775557561562891351E-14, 106.0000000000000000 ) ) ;
#15771=DIRECTION ( 'NONE',  ( -1.000000000000000000, -0.000000000000000000, -0.000000000000000000 ) ) ;
#15797=ORIENTED_EDGE ( 'NONE', *, *, #10595, .T. ) ;
#15804=EDGE_CURVE ( 'NONE', #6257, #52, #21131, .T. ) ;
#15828=ORIENTED_EDGE ( 'NONE', *, *, #32651, .T. ) ;
#15908=AXIS2_PLACEMENT_3D ( 'NONE', #28306, #4189, #6507 ) ;
#15916=ADVANCED_FACE ( 'NONE', ( #137, #33094 ), #311, .F. ) ;
#15930=AXIS2_PLACEMENT_3D ( 'NONE', #11405, #28147, #19656 ) ;
#15936=( NAMED_UNIT ( * ) SI_UNIT ( $, .STERADIAN. ) SOLID_ANGLE_UNIT ( ) );
#15953=DIRECTION ( 'NONE',  ( -0.000000000000000000, -0.000000000000000000, -1.000000000000000000 ) ) ;
#15988=CIRCLE ( 'NONE', #5106, 11.00000000000001066 ) ;
#16003=VERTEX_POINT ( 'NONE', #1035 ) ;
#16009=AXIS2_PLACEMENT_3D ( 'NONE', #23118, #23844, #4240 ) ;
#16013=EDGE_LOOP ( 'NONE', ( #5745, #28484, #7531, #27721 ) ) ;
#16053=VERTEX_POINT ( 'NONE', #835 ) ;
#16058=ORIENTED_EDGE ( 'NONE', *, *, #19802, .T. ) ;
#16063=VERTEX_POINT ( 'NONE', #14507 ) ;
#16070=CARTESIAN_POINT ( 'NONE',  ( -50.00000000000000000, 0.000000000000000000, 64.00000000000000000 ) ) ;
#16090=FACE_BOUND ( 'NONE', #17120, .T. ) ;
#16101=ADVANCED_FACE ( 'NONE', ( #34157 ), #9478, .F. ) ;
#16108=FILL_AREA_STYLE ('',( #32333 ) ) ;
#16127=CARTESIAN_POINT ( 'NONE',  ( -55.00000000000000000, 19.99999999999998934, 110.0000000000000000 ) ) ;
#16148=ORIENTED_EDGE ( 'NONE', *, *, #10570, .F. ) ;
#16166=DIRECTION ( 'NONE',  ( 0.000000000000000000, -1.000000000000000000, 0.000000000000000000 ) ) ;
#16171=CARTESIAN_POINT ( 'NONE',  ( 50.00000000000000000, -25.98076211353320275, 84.99999999999992895 ) ) ;
#16217=AXIS2_PLACEMENT_3D ( 'NONE', #33374, #14448, #6189 ) ;
#16219=VERTEX_POINT ( 'NONE', #21839 ) ;
#16234=EDGE_CURVE ( 'NONE', #9078, #33007, #13753, .T. ) ;
#16255=EDGE_LOOP ( 'NONE', ( #9871, #2562, #13469, #3213 ) ) ;
#16293=CARTESIAN_POINT ( 'NONE',  ( 55.00000000000000000, 10.00000000000000888, 120.0000000000000000 ) ) ;
#16299=CARTESIAN_POINT ( 'NONE',  ( -49.99999999999999289, -25.98076211353320275, 78.99999999999992895 ) ) ;
#16309=CARTESIAN_POINT ( 'NONE',  ( -49.99999999999999289, -25.98076211353320275, 92.99999999999991473 ) ) ;
#16318=ORIENTED_EDGE ( 'NONE', *, *, #5044, .F. ) ;
#16321=DIRECTION ( 'NONE',  ( -1.000000000000000000, -0.000000000000000000, -0.000000000000000000 ) ) ;
#16323=VERTEX_POINT ( 'NONE', #6167 ) ;
#16343=DIRECTION ( 'NONE',  ( 0.000000000000000000, 0.000000000000000000, -1.000000000000000000 ) ) ;
#16347=CARTESIAN_POINT ( 'NONE',  ( -50.00000000000000000, -2.726571689596996976E-14, 114.0000000000000000 ) ) ;
#16359=FACE_BOUND ( 'NONE', #34027, .T. ) ;
#16365=DIRECTION ( 'NONE',  ( 1.000000000000000000, 0.000000000000000000, -0.000000000000000000 ) ) ;
#16371=ORIENTED_EDGE ( 'NONE', *, *, #6168, .F. ) ;
#16400=VECTOR ( 'NONE', #15640, 1000.000000000000000 ) ;
#16405=CARTESIAN_POINT ( 'NONE',  ( 55.00000000000000000, -25.98076211353320275, 84.99999999999994316 ) ) ;
#16439=ADVANCED_FACE ( 'NONE', ( #11569 ), #406, .F. ) ;
#16453=CARTESIAN_POINT ( 'NONE',  ( 55.00000000000000000, 0.000000000000000000, -5.000000000000011546 ) ) ;
#16455=CARTESIAN_POINT ( 'NONE',  ( 46.00000000000000000, 0.000000000000000000, -11.00000000000000000 ) ) ;
#16464=ORIENTED_EDGE ( 'NONE', *, *, #13407, .T. ) ;
#16484=EDGE_CURVE ( 'NONE', #52, #24250, #22710, .T. ) ;
#16503=ORIENTED_EDGE ( 'NONE', *, *, #33687, .T. ) ;
#16506=CARTESIAN_POINT ( 'NONE',  ( -50.00000000000000000, 1.347111479062088405E-15, -11.00000000000000000 ) ) ;
#16509=AXIS2_PLACEMENT_3D ( 'NONE', #24234, #21162, #12897 ) ;
#16520=AXIS2_PLACEMENT_3D ( 'NONE', #13926, #17314, #22906 ) ;
#16524=EDGE_CURVE ( 'NONE', #34014, #30169, #32710, .T. ) ;
#16548=FACE_BOUND ( 'NONE', #28385, .T. ) ;
#16560=DIRECTION ( 'NONE',  ( 1.000000000000000000, -0.000000000000000000, -0.000000000000000000 ) ) ;
#16587=EDGE_LOOP ( 'NONE', ( #7317, #7925, #25622, #11670 ) ) ;
#16594=DIRECTION ( 'NONE',  ( 1.000000000000000000, 0.000000000000000000, 0.000000000000000000 ) ) ;
#16654=AXIS2_PLACEMENT_3D ( 'NONE', #1019, #30723, #28738 ) ;
#16663=CARTESIAN_POINT ( 'NONE',  ( 46.00000000000000000, -25.98076211353320275, 84.99999999999992895 ) ) ;
#16722=EDGE_CURVE ( 'NONE', #26283, #14544, #14290, .T. ) ;
#16767=CARTESIAN_POINT ( 'NONE',  ( -55.00000000000000000, 0.000000000000000000, 64.00000000000000000 ) ) ;
#16796=VERTEX_POINT ( 'NONE', #21840 ) ;
#16803=CIRCLE ( 'NONE', #1297, 10.99999999999999645 ) ;
#16812=DIRECTION ( 'NONE',  ( -1.000000000000000000, -0.000000000000000000, -0.000000000000000000 ) ) ;
#16836=CARTESIAN_POINT ( 'NONE',  ( 50.00000000000000000, 20.00000000000001776, 120.0000000000000000 ) ) ;
#16854=CARTESIAN_POINT ( 'NONE',  ( -46.00000000000000000, 0.000000000000000000, 70.00000000000000000 ) ) ;
#16861=DIRECTION ( 'NONE',  ( 1.000000000000000000, -0.000000000000000000, 0.000000000000000000 ) ) ;
#16903=DIRECTION ( 'NONE',  ( -1.000000000000000000, 0.000000000000000000, 0.000000000000000000 ) ) ;
#16927=EDGE_CURVE ( 'NONE', #24505, #26571, #33533, .T. ) ;
#16932=DIRECTION ( 'NONE',  ( 0.000000000000000000, 0.000000000000000000, -1.000000000000000000 ) ) ;
#16936=VECTOR ( 'NONE', #12660, 1000.000000000000000 ) ;
#16945=ORIENTED_EDGE ( 'NONE', *, *, #1369, .F. ) ;
#16960=DIRECTION ( 'NONE',  ( 1.000000000000000000, -0.000000000000000000, -0.000000000000000000 ) ) ;
#16974=DIRECTION ( 'NONE',  ( 1.000000000000000000, -0.000000000000000000, -0.000000000000000000 ) ) ;
#16989=ORIENTED_EDGE ( 'NONE', *, *, #27573, .T. ) ;
#17044=ORIENTED_EDGE ( 'NONE', *, *, #7697, .T. ) ;
#17065=AXIS2_PLACEMENT_3D ( 'NONE', #20775, #9641, #17910 ) ;
#17070=CARTESIAN_POINT ( 'NONE',  ( -54.99999999999998579, -64.99999999999997158, 120.0000000000000000 ) ) ;
#17083=AXIS2_PLACEMENT_3D ( 'NONE', #3332, #28509, #8704 ) ;
#17088=CIRCLE ( 'NONE', #21099, 11.00000000000001066 ) ;
#17113=ORIENTED_EDGE ( 'NONE', *, *, #7701, .T. ) ;
#17120=EDGE_LOOP ( 'NONE', ( #20390, #23012 ) ) ;
#17151=ORIENTED_EDGE ( 'NONE', *, *, #33395, .F. ) ;
#17154=LINE ( 'NONE', #33733, #2767 ) ;
#17171=CIRCLE ( 'NONE', #10288, 8.000000000000007105 ) ;
#17224=DIRECTION ( 'NONE',  ( 0.000000000000000000, -1.000000000000000000, 0.000000000000000000 ) ) ;
#17266=DIRECTION ( 'NONE',  ( 0.000000000000000000, 0.000000000000000000, 1.000000000000000000 ) ) ;
#17273=DIRECTION ( 'NONE',  ( -1.000000000000000000, -1.734723475976807094E-16, 0.000000000000000000 ) ) ;
#17288=ORIENTED_EDGE ( 'NONE', *, *, #31301, .F. ) ;
#17314=DIRECTION ( 'NONE',  ( -1.000000000000000000, -0.000000000000000000, 0.000000000000000000 ) ) ;
#17315=CIRCLE ( 'NONE', #35168, 5.000000000000011546 ) ;
#17334=ORIENTED_EDGE ( 'NONE', *, *, #24422, .F. ) ;
#17339=ORIENTED_EDGE ( 'NONE', *, *, #10650, .F. ) ;
#17347=EDGE_LOOP ( 'NONE', ( #19177, #810 ) ) ;
#17372=FACE_OUTER_BOUND ( 'NONE', #14253, .T. ) ;
#17373=ORIENTED_EDGE ( 'NONE', *, *, #23577, .T. ) ;
#17398=ORIENTED_EDGE ( 'NONE', *, *, #14093, .T. ) ;
#17440=ORIENTED_EDGE ( 'NONE', *, *, #27606, .F. ) ;
#17445=EDGE_CURVE ( 'NONE', #15308, #11089, #35288, .T. ) ;
#17454=ADVANCED_FACE ( 'NONE', ( #32561 ), #10067, .F. ) ;
#17467=VERTEX_POINT ( 'NONE', #13149 ) ;
#17471=VECTOR ( 'NONE', #18894, 1000.000000000000000 ) ;
#17487=VERTEX_POINT ( 'NONE', #30053 ) ;
#17519=CARTESIAN_POINT ( 'NONE',  ( -46.00000000000000000, -25.98076211353320275, 84.99999999999992895 ) ) ;
#17566=EDGE_CURVE ( 'NONE', #2467, #6941, #28156, .T. ) ;
#17595=AXIS2_PLACEMENT_3D ( 'NONE', #32271, #13366, #7592 ) ;
#17597=ADVANCED_FACE ( 'NONE', ( #8597 ), #8766, .F. ) ;
#17602=DIRECTION ( 'NONE',  ( -1.000000000000000000, 0.000000000000000000, 0.000000000000000000 ) ) ;
#17623=ADVANCED_FACE ( 'NONE', ( #33280 ), #30574, .T. ) ;
#17625=ORIENTED_EDGE ( 'NONE', *, *, #9449, .F. ) ;
#17630=VECTOR ( 'NONE', #9961, 1000.000000000000000 ) ;
#17639=FACE_OUTER_BOUND ( 'NONE', #30503, .T. ) ;
#17647=EDGE_CURVE ( 'NONE', #32025, #2204, #9177, .T. ) ;
#17665=VERTEX_POINT ( 'NONE', #19222 ) ;
#17673=VERTEX_POINT ( 'NONE', #28585 ) ;
#17684=CARTESIAN_POINT ( 'NONE',  ( -55.00000000000000000, -25.98076211353320275, 84.99999999999994316 ) ) ;
#17702=VERTEX_POINT ( 'NONE', #6431 ) ;
#17714=VECTOR ( 'NONE', #28931, 1000.000000000000000 ) ;
#17716=CIRCLE ( 'NONE', #8521, 8.000000000000012434 ) ;
#17735=EDGE_CURVE ( 'NONE', #33969, #26363, #14922, .T. ) ;
#17751=FACE_OUTER_BOUND ( 'NONE', #28175, .T. ) ;
#17752=DIRECTION ( 'NONE',  ( 0.000000000000000000, 0.000000000000000000, 1.000000000000000000 ) ) ;
#17783=DIRECTION ( 'NONE',  ( 1.000000000000000000, -0.000000000000000000, -0.000000000000000000 ) ) ;
#17790=ORIENTED_EDGE ( 'NONE', *, *, #20002, .T. ) ;
#17795=VERTEX_POINT ( 'NONE', #6965 ) ;
#17822=EDGE_CURVE ( 'NONE', #16219, #12018, #31630, .T. ) ;
#17845=VERTEX_POINT ( 'NONE', #28403 ) ;
#17847=DIRECTION ( 'NONE',  ( -1.000000000000000000, -1.734723475976807094E-16, -0.000000000000000000 ) ) ;
#17848=PRODUCT ( 'Mounting Base Plate Frame', 'Mounting Base Plate Frame', '', ( #33801 ) ) ;
#17864=EDGE_CURVE ( 'NONE', #5260, #16053, #5039, .T. ) ;
#17892=EDGE_CURVE ( 'NONE', #32586, #17665, #29764, .T. ) ;
#17903=DIRECTION ( 'NONE',  ( 0.000000000000000000, 0.000000000000000000, 1.000000000000000000 ) ) ;
#17908=EDGE_CURVE ( 'NONE', #17702, #5884, #18482, .T. ) ;
#17910=DIRECTION ( 'NONE',  ( 1.734723475976807094E-16, -1.000000000000000000, 0.000000000000000000 ) ) ;
#17916=AXIS2_PLACEMENT_3D ( 'NONE', #10301, #21262, #32262 ) ;
#17919=FACE_OUTER_BOUND ( 'NONE', #31974, .T. ) ;
#17936=LINE ( 'NONE', #7140, #7024 ) ;
#17939=ORIENTED_EDGE ( 'NONE', *, *, #18521, .T. ) ;
#18073=EDGE_CURVE ( 'NONE', #16796, #6343, #29224, .T. ) ;
#18104=CIRCLE ( 'NONE', #2612, 11.00000000000001066 ) ;
#18111=VERTEX_POINT ( 'NONE', #16293 ) ;
#18133=( LENGTH_UNIT ( ) NAMED_UNIT ( * ) SI_UNIT ( .MILLI., .METRE. ) );
#18159=APPLICATION_CONTEXT ( 'automotive_design' ) ;
#18185=ORIENTED_EDGE ( 'NONE', *, *, #18732, .T. ) ;
#18194=AXIS2_PLACEMENT_3D ( 'NONE', #20146, #28639, #23409 ) ;
#18201=ADVANCED_FACE ( 'NONE', ( #13618, #10925 ), #21892, .T. ) ;
#18214=VECTOR ( 'NONE', #31958, 1000.000000000000000 ) ;
#18216=DIRECTION ( 'NONE',  ( 1.000000000000000000, 0.000000000000000000, 0.000000000000000000 ) ) ;
#18221=AXIS2_PLACEMENT_3D ( 'NONE', #14090, #238, #19494 ) ;
#18226=ORIENTED_EDGE ( 'NONE', *, *, #31545, .T. ) ;
#18227=VECTOR ( 'NONE', #27070, 1000.000000000000000 ) ;
#18264=DIRECTION ( 'NONE',  ( 1.000000000000000000, -0.000000000000000000, -0.000000000000000000 ) ) ;
#18272=LINE ( 'NONE', #15199, #4641 ) ;
#18292=DIRECTION ( 'NONE',  ( 1.000000000000000000, 0.000000000000000000, 0.000000000000000000 ) ) ;
#18294=VERTEX_POINT ( 'NONE', #31237 ) ;
#18304=EDGE_CURVE ( 'NONE', #32416, #1635, #8537, .T. ) ;
#18329=LINE ( 'NONE', #10422, #7707 ) ;
#18366=ORIENTED_EDGE ( 'NONE', *, *, #24422, .T. ) ;
#18389=EDGE_LOOP ( 'NONE', ( #14407, #3869, #10623, #14235 ) ) ;
#18408=AXIS2_PLACEMENT_3D ( 'NONE', #22066, #27493, #25132 ) ;
#18413=AXIS2_PLACEMENT_3D ( 'NONE', #34775, #10097, #27032 ) ;
#18423=DIRECTION ( 'NONE',  ( 0.000000000000000000, 0.000000000000000000, -1.000000000000000000 ) ) ;
#18451=CARTESIAN_POINT ( 'NONE',  ( -46.00000000000000000, 0.000000000000000000, 8.000000000000000000 ) ) ;
#18462=ORIENTED_EDGE ( 'NONE', *, *, #27573, .F. ) ;
#18469=CARTESIAN_POINT ( 'NONE',  ( 55.00000000000000000, 20.00000000000001776, 110.0000000000000000 ) ) ;
#18482=LINE ( 'NONE', #15761, #12503 ) ;
#18505=ORIENTED_EDGE ( 'NONE', *, *, #35480, .F. ) ;
#18516=EDGE_LOOP ( 'NONE', ( #4309, #32409 ) ) ;
#18517=ORIENTED_EDGE ( 'NONE', *, *, #27868, .F. ) ;
#18521=EDGE_CURVE ( 'NONE', #17673, #35062, #11010, .T. ) ;
#18563=EDGE_LOOP ( 'NONE', ( #34569, #32081, #32790, #3426 ) ) ;
#18567=CIRCLE ( 'NONE', #20262, 11.00000000000000000 ) ;
#18580=AXIS2_PLACEMENT_3D ( 'NONE', #10959, #22104, #33100 ) ;
#18597=ADVANCED_FACE ( 'NONE', ( #22329 ), #33150, .F. ) ;
#18679=EDGE_CURVE ( 'NONE', #16323, #30634, #3620, .T. ) ;
#18693=VECTOR ( 'NONE', #20261, 1000.000000000000000 ) ;
#18694=CARTESIAN_POINT ( 'NONE',  ( -55.00000000000000000, 0.000000000000000000, 0.000000000000000000 ) ) ;
#18702=CARTESIAN_POINT ( 'NONE',  ( -46.00000000000000000, 0.000000000000000000, 70.00000000000000000 ) ) ;
#18732=EDGE_CURVE ( 'NONE', #12018, #35000, #25209, .T. ) ;
#18738=AXIS2_PLACEMENT_3D ( 'NONE', #5110, #7600, #29589 ) ;
#18752=CARTESIAN_POINT ( 'NONE',  ( -49.99999999999998579, -60.00000000000000000, 120.0000000000000000 ) ) ;
#18753=DIRECTION ( 'NONE',  ( -1.000000000000000000, 0.000000000000000000, 0.000000000000000000 ) ) ;
#18789=AXIS2_PLACEMENT_3D ( 'NONE', #30060, #21938, #19229 ) ;
#18814=LINE ( 'NONE', #13594, #20992 ) ;
#18848=AXIS2_PLACEMENT_3D ( 'NONE', #20662, #6821, #15264 ) ;
#18854=ORIENTED_EDGE ( 'NONE', *, *, #17566, .T. ) ;
#18869=AXIS2_PLACEMENT_3D ( 'NONE', #1743, #12547, #34514 ) ;
#18876=DIRECTION ( 'NONE',  ( 1.000000000000000000, -0.000000000000000000, -0.000000000000000000 ) ) ;
#18890=DIRECTION ( 'NONE',  ( 1.000000000000000000, 1.734723475976807094E-16, -0.000000000000000000 ) ) ;
#18894=DIRECTION ( 'NONE',  ( -0.000000000000000000, -1.000000000000000000, 0.000000000000000000 ) ) ;
#18905=CARTESIAN_POINT ( 'NONE',  ( -55.00000000000000000, -2.726571689596996976E-14, 114.0000000000000000 ) ) ;
#18909=CYLINDRICAL_SURFACE ( 'NONE', #18413, 11.00000000000000000 ) ;
#18912=ORIENTED_EDGE ( 'NONE', *, *, #24504, .F. ) ;
#18913=CARTESIAN_POINT ( 'NONE',  ( -50.00000000000000000, 0.000000000000000000, 0.000000000000000000 ) ) ;
#18924=ADVANCED_FACE ( 'NONE', ( #5226 ), #21400, .T. ) ;
#18932=CARTESIAN_POINT ( 'NONE',  ( -55.00000000000000000, 10.00000000000000888, 110.0000000000000000 ) ) ;
#18934=EDGE_CURVE ( 'NONE', #4303, #28364, #26942, .T. ) ;
#18971=DIRECTION ( 'NONE',  ( 1.000000000000000000, 0.000000000000000000, 0.000000000000000000 ) ) ;
#18979=AXIS2_PLACEMENT_3D ( 'NONE', #11163, #8274, #32953 ) ;
#19018=ADVANCED_FACE ( 'NONE', ( #28927 ), #9476, .T. ) ;
#19021=FACE_BOUND ( 'NONE', #3743, .T. ) ;
#19029=VERTEX_POINT ( 'NONE', #6957 ) ;
#19052=ORIENTED_EDGE ( 'NONE', *, *, #11253, .T. ) ;
#19097=VECTOR ( 'NONE', #31899, 1000.000000000000000 ) ;
#19135=ADVANCED_FACE ( 'NONE', ( #17751 ), #1564, .F. ) ;
#19147=CIRCLE ( 'NONE', #22031, 10.00000000000000000 ) ;
#19162=DIRECTION ( 'NONE',  ( -1.000000000000000000, 0.000000000000000000, 0.000000000000000000 ) ) ;
#19177=ORIENTED_EDGE ( 'NONE', *, *, #7697, .F. ) ;
#19189=CARTESIAN_POINT ( 'NONE',  ( -50.00000000000000000, 19.99999999999998934, 120.0000000000000000 ) ) ;
#19190=DIRECTION ( 'NONE',  ( -1.000000000000000000, -0.000000000000000000, 0.000000000000000000 ) ) ;
#19208=EDGE_LOOP ( 'NONE', ( #21380, #18226, #24067, #22782, #9879, #28045, #5203, #17625 ) ) ;
#19222=CARTESIAN_POINT ( 'NONE',  ( 50.00000000000000000, 9.797174393178825657E-16, 8.000000000000000000 ) ) ;
#19229=DIRECTION ( 'NONE',  ( 0.000000000000000000, 0.000000000000000000, -1.000000000000000000 ) ) ;
#19230=ADVANCED_FACE ( 'NONE', ( #27488 ), #13271, .F. ) ;
#19241=FACE_BOUND ( 'NONE', #23099, .T. ) ;
#19244=CLOSED_SHELL ( 'NONE', ( #2866, #10402, #24391, #4457, #10380, #22326, #11412, #31116, #28190, #29801, #6244, #1136, #28439, #23407, #29472, #23074, #19397, #16439, #29009, #18597, #23265, #15916, #29263, #13617, #1530, #12565, #4239, #26674, #11276, #35098, #27835, #4208, #14205, #19875, #15211, #239, #11221, #30159, #17623, #19018, #24480, #31460, #19230, #5378, #29664, #30841, #17454, #35023, #7069, #30995, #30033, #30999, #35329, #17597, #18201, #18924, #7582, #20553, #34597, #8237, #1912, #24229, #19135, #29717, #6198, #16101, #28397, #34516, #27525 ) ) ;
#19251=AXIS2_PLACEMENT_3D ( 'NONE', #33604, #12008, #18423 ) ;
#19260=VERTEX_POINT ( 'NONE', #24603 ) ;
#19273=VECTOR ( 'NONE', #30514, 1000.000000000000000 ) ;
#19276=DIRECTION ( 'NONE',  ( 0.000000000000000000, 0.000000000000000000, -1.000000000000000000 ) ) ;
#19287=DIRECTION ( 'NONE',  ( 0.000000000000000000, -0.000000000000000000, 1.000000000000000000 ) ) ;
#19292=CARTESIAN_POINT ( 'NONE',  ( -55.00000000000000000, -2.775557561562891351E-14, 110.0000000000000000 ) ) ;
#19300=ORIENTED_EDGE ( 'NONE', *, *, #32651, .F. ) ;
#19304=AXIS2_PLACEMENT_3D ( 'NONE', #22219, #16812, #3157 ) ;
#19339=DIRECTION ( 'NONE',  ( 1.000000000000000000, -0.000000000000000000, -0.000000000000000000 ) ) ;
#19365=CARTESIAN_POINT ( 'NONE',  ( -55.00000000000000000, -25.98076211353320275, 90.99999999999994316 ) ) ;
#19372=DIRECTION ( 'NONE',  ( 1.000000000000000000, 0.000000000000000000, -0.000000000000000000 ) ) ;
#19397=ADVANCED_FACE ( 'NONE', ( #11258 ), #19861, .F. ) ;
#19405=CARTESIAN_POINT ( 'NONE',  ( -50.00000000000000000, 19.99999999999998934, 110.0000000000000000 ) ) ;
#19420=AXIS2_PLACEMENT_3D ( 'NONE', #26265, #17602, #32020 ) ;
#19435=ORIENTED_EDGE ( 'NONE', *, *, #11982, .T. ) ;
#19494=DIRECTION ( 'NONE',  ( 0.000000000000000000, 0.000000000000000000, -1.000000000000000000 ) ) ;
#19506=CARTESIAN_POINT ( 'NONE',  ( 50.00000000000000000, 0.000000000000000000, 61.99999999999999289 ) ) ;
#19508=CARTESIAN_POINT ( 'NONE',  ( -55.00000000000000000, 7.347880794884119736E-16, 76.00000000000001421 ) ) ;
#19510=VECTOR ( 'NONE', #29584, 1000.000000000000000 ) ;
#19518=VERTEX_POINT ( 'NONE', #23710 ) ;
#19528=AXIS2_PLACEMENT_3D ( 'NONE', #3906, #19886, #22596 ) ;
#19562=ORIENTED_EDGE ( 'NONE', *, *, #26966, .F. ) ;
#19574=AXIS2_PLACEMENT_3D ( 'NONE', #33169, #21459, #5635 ) ;
#19602=EDGE_CURVE ( 'NONE', #8628, #5884, #22375, .T. ) ;
#19622=ORIENTED_EDGE ( 'NONE', *, *, #15581, .F. ) ;
#19629=EDGE_LOOP ( 'NONE', ( #21010, #1979 ) ) ;
#19648=ORIENTED_EDGE ( 'NONE', *, *, #13427, .F. ) ;
#19656=DIRECTION ( 'NONE',  ( 0.000000000000000000, 0.000000000000000000, -1.000000000000000000 ) ) ;
#19660=CIRCLE ( 'NONE', #16217, 0.9999999999999974465 ) ;
#19671=CIRCLE ( 'NONE', #5350, 6.000000000000005329 ) ;
#19679=LINE ( 'NONE', #22927, #25758 ) ;
#19698=FACE_BOUND ( 'NONE', #30264, .T. ) ;
#19701=DIRECTION ( 'NONE',  ( -1.000000000000000000, -0.000000000000000000, -0.000000000000000000 ) ) ;
#19734=DIRECTION ( 'NONE',  ( 1.000000000000000000, -0.000000000000000000, -0.000000000000000000 ) ) ;
#19741=DIRECTION ( 'NONE',  ( 0.000000000000000000, -1.000000000000000000, 0.000000000000000000 ) ) ;
#19802=EDGE_CURVE ( 'NONE', #20350, #33969, #5694, .T. ) ;
#19838=CARTESIAN_POINT ( 'NONE',  ( 50.00000000000000000, 1.347111479062090574E-15, 81.00000000000001421 ) ) ;
#19861=CYLINDRICAL_SURFACE ( 'NONE', #6836, 6.000000000000005329 ) ;
#19875=ADVANCED_FACE ( 'NONE', ( #6040, #461, #30364, #25307, #13966 ), #24957, .F. ) ;
#19876=FACE_OUTER_BOUND ( 'NONE', #28916, .T. ) ;
#19886=DIRECTION ( 'NONE',  ( -1.000000000000000000, -0.000000000000000000, -0.000000000000000000 ) ) ;
#19892=AXIS2_PLACEMENT_3D ( 'NONE', #35123, #15281, #26296 ) ;
#19918=CIRCLE ( 'NONE', #16520, 9.999999999999994671 ) ;
#19923=AXIS2_PLACEMENT_3D ( 'NONE', #20098, #3744, #26064 ) ;
#19924=CIRCLE ( 'NONE', #14749, 8.000000000000000000 ) ;
#19941=CARTESIAN_POINT ( 'NONE',  ( 46.00000000000000000, 0.000000000000000000, 0.000000000000000000 ) ) ;
#19958=CARTESIAN_POINT ( 'NONE',  ( 50.00000000000000000, 0.000000000000000000, 70.00000000000000000 ) ) ;
#19975=ORIENTED_EDGE ( 'NONE', *, *, #26088, .F. ) ;
#19978=FACE_OUTER_BOUND ( 'NONE', #651, .T. ) ;
#19990=DIRECTION ( 'NONE',  ( 1.734723475976807094E-16, -1.000000000000000000, 0.000000000000000000 ) ) ;
#20002=EDGE_CURVE ( 'NONE', #10849, #10711, #15489, .T. ) ;
#20004=ORIENTED_EDGE ( 'NONE', *, *, #1871, .T. ) ;
#20036=DIRECTION ( 'NONE',  ( 1.000000000000000000, 0.000000000000000000, 0.000000000000000000 ) ) ;
#20061=STYLED_ITEM ( 'NONE', ( #15597 ), #10186 ) ;
#20064=CARTESIAN_POINT ( 'NONE',  ( 55.00000000000000000, 10.00000000000000888, -15.00000000000000178 ) ) ;
#20098=CARTESIAN_POINT ( 'NONE',  ( 50.00000000000000000, 0.000000000000000000, 70.00000000000000000 ) ) ;
#20124=DIRECTION ( 'NONE',  ( 0.000000000000000000, 0.000000000000000000, 1.000000000000000000 ) ) ;
#20138=CIRCLE ( 'NONE', #35147, 8.000000000000000000 ) ;
#20146=CARTESIAN_POINT ( 'NONE',  ( 46.00000000000000000, -25.98076211353320275, 84.99999999999992895 ) ) ;
#20148=DIRECTION ( 'NONE',  ( 0.000000000000000000, 0.000000000000000000, 1.000000000000000000 ) ) ;
#20203=FACE_OUTER_BOUND ( 'NONE', #20796, .T. ) ;
#20261=DIRECTION ( 'NONE',  ( -1.000000000000000000, -0.000000000000000000, -0.000000000000000000 ) ) ;
#20262=AXIS2_PLACEMENT_3D ( 'NONE', #27187, #32224, #7719 ) ;
#20268=DIRECTION ( 'NONE',  ( 1.000000000000000000, -0.000000000000000000, -0.000000000000000000 ) ) ;
#20273=AXIS2_PLACEMENT_3D ( 'NONE', #18694, #27534, #13485 ) ;
#20316=EDGE_CURVE ( 'NONE', #29062, #15120, #10939, .T. ) ;
#20338=DIRECTION ( 'NONE',  ( 1.000000000000000000, 0.000000000000000000, 0.000000000000000000 ) ) ;
#20350=VERTEX_POINT ( 'NONE', #2963 ) ;
#20360=CARTESIAN_POINT ( 'NONE',  ( 50.00000000000000000, 10.00000000000000888, 120.0000000000000000 ) ) ;
#20370=DIRECTION ( 'NONE',  ( 1.000000000000000000, -0.000000000000000000, -0.000000000000000000 ) ) ;
#20390=ORIENTED_EDGE ( 'NONE', *, *, #33326, .T. ) ;
#20402=CARTESIAN_POINT ( 'NONE',  ( 46.00000000000000000, -25.98076211353320275, 95.99999999999991473 ) ) ;
#20405=UNCERTAINTY_MEASURE_WITH_UNIT (LENGTH_MEASURE( 1.000000000000000082E-05 ), #18133, 'distance_accuracy_value', 'NONE');
#20435=CARTESIAN_POINT ( 'NONE',  ( -46.00000000000000000, 0.000000000000000000, 70.00000000000000000 ) ) ;
#20440=ORIENTED_EDGE ( 'NONE', *, *, #16524, .T. ) ;
#20442=AXIS2_PLACEMENT_3D ( 'NONE', #25334, #299, #27854 ) ;
#20448=EDGE_LOOP ( 'NONE', ( #11090, #13306 ) ) ;
#20484=CYLINDRICAL_SURFACE ( 'NONE', #18848, 11.00000000000001066 ) ;
#20526=ORIENTED_EDGE ( 'NONE', *, *, #20697, .F. ) ;
#20527=VECTOR ( 'NONE', #8866, 1000.000000000000000 ) ;
#20553=ADVANCED_FACE ( 'NONE', ( #6435, #11486 ), #6263, .T. ) ;
#20638=LINE ( 'NONE', #29659, #32031 ) ;
#20658=ORIENTED_EDGE ( 'NONE', *, *, #16927, .F. ) ;
#20662=CARTESIAN_POINT ( 'NONE',  ( -46.00000000000000000, 0.000000000000000000, 70.00000000000000000 ) ) ;
#20666=EDGE_CURVE ( 'NONE', #28349, #11089, #616, .T. ) ;
#20671=CARTESIAN_POINT ( 'NONE',  ( -55.00000000000000000, 0.000000000000000000, 70.00000000000000000 ) ) ;
#20672=AXIS2_PLACEMENT_3D ( 'NONE', #7097, #12151, #20943 ) ;
#20684=CYLINDRICAL_SURFACE ( 'NONE', #18194, 7.999999999999992895 ) ;
#20685=EDGE_CURVE ( 'NONE', #2539, #16003, #8095, .T. ) ;
#20687=ORIENTED_EDGE ( 'NONE', *, *, #5817, .F. ) ;
#20697=EDGE_CURVE ( 'NONE', #30657, #16063, #32833, .T. ) ;
#20749=CARTESIAN_POINT ( 'NONE',  ( 46.00000000000000000, -25.98076211353320275, 84.99999999999992895 ) ) ;
#20775=CARTESIAN_POINT ( 'NONE',  ( -50.00000000000000000, 19.99999999999998934, 120.0000000000000000 ) ) ;
#20779=DIRECTION ( 'NONE',  ( -1.000000000000000000, -1.734723475976807094E-16, 0.000000000000000000 ) ) ;
#20780=DIRECTION ( 'NONE',  ( -1.000000000000000000, -0.000000000000000000, -0.000000000000000000 ) ) ;
#20796=EDGE_LOOP ( 'NONE', ( #15797, #6241, #18912, #6843 ) ) ;
#20798=CARTESIAN_POINT ( 'NONE',  ( -50.00000000000000000, 19.99999999999998934, 110.0000000000000000 ) ) ;
#20801=EDGE_LOOP ( 'NONE', ( #22853, #33967, #35302, #4861, #6008, #10045 ) ) ;
#20808=DIRECTION ( 'NONE',  ( 0.000000000000000000, 0.000000000000000000, -1.000000000000000000 ) ) ;
#20818=DIRECTION ( 'NONE',  ( 1.000000000000000000, -0.000000000000000000, -0.000000000000000000 ) ) ;
#20819=CARTESIAN_POINT ( 'NONE',  ( -29.99999999999999645, -26.99999999999999645, 113.9999999999999858 ) ) ;
#20820=FILL_AREA_STYLE ('',( #31824 ) ) ;
#20871=CIRCLE ( 'NONE', #11681, 10.99999999999999645 ) ;
#20882=AXIS2_PLACEMENT_3D ( 'NONE', #8729, #21896, #14140 ) ;
#20892=CIRCLE ( 'NONE', #9416, 4.000000000000003553 ) ;
#20913=DIRECTION ( 'NONE',  ( 1.000000000000000000, 0.000000000000000000, 0.000000000000000000 ) ) ;
#20915=ORIENTED_EDGE ( 'NONE', *, *, #25997, .T. ) ;
#20918=CARTESIAN_POINT ( 'NONE',  ( -50.00000000000000000, 1.347111479062090574E-15, 59.00000000000000000 ) ) ;
#20943=DIRECTION ( 'NONE',  ( 0.000000000000000000, 0.000000000000000000, -1.000000000000000000 ) ) ;
#20966=ORIENTED_EDGE ( 'NONE', *, *, #34052, .F. ) ;
#20991=EDGE_CURVE ( 'NONE', #33007, #19518, #8211, .T. ) ;
#20992=VECTOR ( 'NONE', #35220, 1000.000000000000000 ) ;
#21010=ORIENTED_EDGE ( 'NONE', *, *, #678, .F. ) ;
#21027=ORIENTED_EDGE ( 'NONE', *, *, #3429, .F. ) ;
#21031=DIRECTION ( 'NONE',  ( 0.000000000000000000, 0.000000000000000000, 1.000000000000000000 ) ) ;
#21099=AXIS2_PLACEMENT_3D ( 'NONE', #14034, #21785, #3253 ) ;
#21103=VECTOR ( 'NONE', #13247, 1000.000000000000000 ) ;
#21125=VECTOR ( 'NONE', #33662, 1000.000000000000000 ) ;
#21131=CIRCLE ( 'NONE', #23458, 0.9999999999999974465 ) ;
#21139=ORIENTED_EDGE ( 'NONE', *, *, #3525, .F. ) ;
#21143=PLANE ( 'NONE',  #35386 ) ;
#21154=AXIS2_PLACEMENT_3D ( 'NONE', #32884, #5519, #9273 ) ;
#21162=DIRECTION ( 'NONE',  ( -1.000000000000000000, 0.000000000000000000, 0.000000000000000000 ) ) ;
#21200=DIRECTION ( 'NONE',  ( 0.000000000000000000, 0.000000000000000000, 1.000000000000000000 ) ) ;
#21223=DIRECTION ( 'NONE',  ( 0.000000000000000000, 0.000000000000000000, -1.000000000000000000 ) ) ;
#21242=VERTEX_POINT ( 'NONE', #20402 ) ;
#21254=ORIENTED_EDGE ( 'NONE', *, *, #7535, .F. ) ;
#21262=DIRECTION ( 'NONE',  ( -1.000000000000000000, -0.000000000000000000, -0.000000000000000000 ) ) ;
#21264=PRODUCT_DEFINITION_FORMATION_WITH_SPECIFIED_SOURCE ( 'ANY', '', #17848, .NOT_KNOWN. ) ;
#21268=DIRECTION ( 'NONE',  ( 1.000000000000000000, -0.000000000000000000, -0.000000000000000000 ) ) ;
#21273=CARTESIAN_POINT ( 'NONE',  ( -49.99999999999998579, -60.00000000000000000, 120.0000000000000000 ) ) ;
#21284=DIRECTION ( 'NONE',  ( 1.000000000000000000, -0.000000000000000000, -0.000000000000000000 ) ) ;
#21289=ORIENTED_EDGE ( 'NONE', *, *, #17445, .T. ) ;
#21298=ORIENTED_EDGE ( 'NONE', *, *, #10848, .F. ) ;
#21306=VECTOR ( 'NONE', #21284, 1000.000000000000000 ) ;
#21307=AXIS2_PLACEMENT_3D ( 'NONE', #26589, #12725, #18292 ) ;
#21308=AXIS2_PLACEMENT_3D ( 'NONE', #29737, #13352, #35499 ) ;
#21312=EDGE_CURVE ( 'NONE', #23442, #26801, #25854, .T. ) ;
#21379=DIRECTION ( 'NONE',  ( -1.000000000000000000, -0.000000000000000000, -0.000000000000000000 ) ) ;
#21380=ORIENTED_EDGE ( 'NONE', *, *, #24916, .F. ) ;
#21400=CYLINDRICAL_SURFACE ( 'NONE', #2791, 11.00000000000001066 ) ;
#21435=EDGE_CURVE ( 'NONE', #33466, #17702, #9974, .T. ) ;
#21436=CIRCLE ( 'NONE', #22001, 9.999999999999994671 ) ;
#21447=VECTOR ( 'NONE', #8763, 1000.000000000000000 ) ;
#21454=EDGE_LOOP ( 'NONE', ( #23607, #4772, #26060, #1456 ) ) ;
#21459=DIRECTION ( 'NONE',  ( 0.000000000000000000, 0.000000000000000000, -1.000000000000000000 ) ) ;
#21499=EDGE_LOOP ( 'NONE', ( #32230, #33483 ) ) ;
#21522=CIRCLE ( 'NONE', #25589, 6.000000000000005329 ) ;
#21535=CYLINDRICAL_SURFACE ( 'NONE', #34905, 5.000000000000011546 ) ;
#21537=DIRECTION ( 'NONE',  ( 0.000000000000000000, 0.000000000000000000, 1.000000000000000000 ) ) ;
#21569=DIRECTION ( 'NONE',  ( -1.000000000000000000, -1.734723475976807094E-16, 0.000000000000000000 ) ) ;
#21580=ORIENTED_EDGE ( 'NONE', *, *, #269, .F. ) ;
#21620=DIRECTION ( 'NONE',  ( -1.000000000000000000, -1.387778780781445922E-16, -0.000000000000000000 ) ) ;
#21660=VECTOR ( 'NONE', #16960, 1000.000000000000000 ) ;
#21669=CIRCLE ( 'NONE', #6715, 8.000000000000000000 ) ;
#21675=CARTESIAN_POINT ( 'NONE',  ( -49.99999999999998579, -60.00000000000000000, -25.00000000000000000 ) ) ;
#21676=CARTESIAN_POINT ( 'NONE',  ( 46.00000000000000000, 0.000000000000000000, -8.000000000000000000 ) ) ;
#21700=( NAMED_UNIT ( * ) PLANE_ANGLE_UNIT ( ) SI_UNIT ( $, .RADIAN. ) );
#21709=DIRECTION ( 'NONE',  ( -1.000000000000000000, -1.734723475976807094E-16, 0.000000000000000000 ) ) ;
#21726=ORIENTED_EDGE ( 'NONE', *, *, #14808, .F. ) ;
#21733=DIRECTION ( 'NONE',  ( -1.000000000000000000, 0.000000000000000000, 0.000000000000000000 ) ) ;
#21738=PLANE ( 'NONE',  #851 ) ;
#21742=DIRECTION ( 'NONE',  ( 1.000000000000000000, -0.000000000000000000, -0.000000000000000000 ) ) ;
#21749=AXIS2_PLACEMENT_3D ( 'NONE', #24280, #21733, #27333 ) ;
#21785=DIRECTION ( 'NONE',  ( -1.000000000000000000, 0.000000000000000000, 0.000000000000000000 ) ) ;
#21800=MECHANICAL_DESIGN_GEOMETRIC_PRESENTATION_REPRESENTATION('',(#20061),#6288);
#21839=CARTESIAN_POINT ( 'NONE',  ( -46.00000000000000000, 0.000000000000000000, 78.00000000000001421 ) ) ;
#21840=CARTESIAN_POINT ( 'NONE',  ( -46.00000000000000000, -25.98076211353320275, 73.99999999999992895 ) ) ;
#21869=LINE ( 'NONE', #4627, #28543 ) ;
#21873=CARTESIAN_POINT ( 'NONE',  ( 46.00000000000000000, -25.98076211353320275, 73.99999999999992895 ) ) ;
#21885=AXIS2_PLACEMENT_3D ( 'NONE', #28094, #25033, #14554 ) ;
#21892=PLANE ( 'NONE',  #21154 ) ;
#21896=DIRECTION ( 'NONE',  ( 1.000000000000000000, 0.000000000000000000, -0.000000000000000000 ) ) ;
#21917=ORIENTED_EDGE ( 'NONE', *, *, #17892, .T. ) ;
#21929=ORIENTED_EDGE ( 'NONE', *, *, #23774, .T. ) ;
#21938=DIRECTION ( 'NONE',  ( -1.000000000000000000, -0.000000000000000000, 0.000000000000000000 ) ) ;
#21944=VERTEX_POINT ( 'NONE', #24001 ) ;
#21989=EDGE_LOOP ( 'NONE', ( #15663, #8272 ) ) ;
#21992=EDGE_LOOP ( 'NONE', ( #11169, #4889 ) ) ;
#22000=CARTESIAN_POINT ( 'NONE',  ( -49.99999999999999289, -25.98076211353320275, 76.99999999999992895 ) ) ;
#22001=AXIS2_PLACEMENT_3D ( 'NONE', #22915, #250, #25634 ) ;
#22024=EDGE_CURVE ( 'NONE', #16053, #5260, #25668, .T. ) ;
#22031=AXIS2_PLACEMENT_3D ( 'NONE', #33066, #19190, #467 ) ;
#22055=EDGE_LOOP ( 'NONE', ( #21139, #27856, #31311, #6360 ) ) ;
#22056=EDGE_CURVE ( 'NONE', #17845, #24505, #32443, .T. ) ;
#22065=CIRCLE ( 'NONE', #10062, 11.00000000000000000 ) ;
#22066=CARTESIAN_POINT ( 'NONE',  ( 50.00000000000000000, 20.00000000000001776, 120.0000000000000000 ) ) ;
#22092=ORIENTED_EDGE ( 'NONE', *, *, #14474, .F. ) ;
#22094=CARTESIAN_POINT ( 'NONE',  ( -46.00000000000000000, 0.000000000000000000, 0.000000000000000000 ) ) ;
#22098=DIRECTION ( 'NONE',  ( 0.000000000000000000, 0.000000000000000000, 1.000000000000000000 ) ) ;
#22103=AXIS2_PLACEMENT_3D ( 'NONE', #9687, #20818, #22824 ) ;
#22104=DIRECTION ( 'NONE',  ( 1.000000000000000000, 0.000000000000000000, -0.000000000000000000 ) ) ;
#22161=ORIENTED_EDGE ( 'NONE', *, *, #21435, .T. ) ;
#22180=AXIS2_PLACEMENT_3D ( 'NONE', #15245, #1236, #9331 ) ;
#22198=CARTESIAN_POINT ( 'NONE',  ( -46.00000000000000000, 0.000000000000000000, 0.000000000000000000 ) ) ;
#22219=CARTESIAN_POINT ( 'NONE',  ( -46.00000000000000000, -25.98076211353320275, 84.99999999999992895 ) ) ;
#22237=AXIS2_PLACEMENT_3D ( 'NONE', #26324, #3828, #29014 ) ;
#22239=CARTESIAN_POINT ( 'NONE',  ( 50.00000000000000000, 20.00000000000001776, 120.0000000000000000 ) ) ;
#22272=FACE_OUTER_BOUND ( 'NONE', #23840, .T. ) ;
#22300=ORIENTED_EDGE ( 'NONE', *, *, #788, .F. ) ;
#22318=CIRCLE ( 'NONE', #26954, 8.000000000000000000 ) ;
#22321=EDGE_LOOP ( 'NONE', ( #3032, #10487 ) ) ;
#22324=ORIENTED_EDGE ( 'NONE', *, *, #16722, .T. ) ;
#22326=ADVANCED_FACE ( 'NONE', ( #17639 ), #22864, .T. ) ;
#22329=FACE_OUTER_BOUND ( 'NONE', #11739, .T. ) ;
#22338=VERTEX_POINT ( 'NONE', #32754 ) ;
#22348=CARTESIAN_POINT ( 'NONE',  ( -50.00000000000000000, 0.000000000000000000, 0.000000000000000000 ) ) ;
#22353=ORIENTED_EDGE ( 'NONE', *, *, #33936, .F. ) ;
#22361=DIRECTION ( 'NONE',  ( 1.000000000000000000, -0.000000000000000000, -0.000000000000000000 ) ) ;
#22369=LINE ( 'NONE', #33899, #21660 ) ;
#22375=CIRCLE ( 'NONE', #32164, 4.000000000000006217 ) ;
#22400=ORIENTED_EDGE ( 'NONE', *, *, #13439, .T. ) ;
#22407=DIRECTION ( 'NONE',  ( -0.000000000000000000, 0.000000000000000000, -1.000000000000000000 ) ) ;
#22502=CARTESIAN_POINT ( 'NONE',  ( -55.00000000000000000, -25.98076211353320275, 84.99999999999994316 ) ) ;
#22528=CYLINDRICAL_SURFACE ( 'NONE', #25678, 4.000000000000003553 ) ;
#22541=ORIENTED_EDGE ( 'NONE', *, *, #10206, .F. ) ;
#22556=CARTESIAN_POINT ( 'NONE',  ( 50.00000000000000000, -25.98076211353320275, 73.99999999999992895 ) ) ;
#22596=DIRECTION ( 'NONE',  ( 0.000000000000000000, 0.000000000000000000, 1.000000000000000000 ) ) ;
#22622=DIRECTION ( 'NONE',  ( 1.000000000000000000, -0.000000000000000000, 0.000000000000000000 ) ) ;
#22625=DIRECTION ( 'NONE',  ( -1.000000000000000000, 0.000000000000000000, 0.000000000000000000 ) ) ;
#22646=EDGE_CURVE ( 'NONE', #11697, #32964, #4788, .T. ) ;
#22654=CYLINDRICAL_SURFACE ( 'NONE', #34966, 4.000000000000003553 ) ;
#22656=ORIENTED_EDGE ( 'NONE', *, *, #19602, .F. ) ;
#22661=AXIS2_PLACEMENT_3D ( 'NONE', #31299, #14721, #34187 ) ;
#22670=CARTESIAN_POINT ( 'NONE',  ( 50.00000000000000000, 20.00000000000001776, 120.0000000000000000 ) ) ;
#22702=ORIENTED_EDGE ( 'NONE', *, *, #2260, .F. ) ;
#22703=VERTEX_POINT ( 'NONE', #21676 ) ;
#22710=LINE ( 'NONE', #9042, #29272 ) ;
#22716=ORIENTED_EDGE ( 'NONE', *, *, #28565, .T. ) ;
#22739=DIRECTION ( 'NONE',  ( 1.000000000000000000, -0.000000000000000000, -0.000000000000000000 ) ) ;
#22742=EDGE_CURVE ( 'NONE', #52, #6257, #19660, .T. ) ;
#22745=VERTEX_POINT ( 'NONE', #19838 ) ;
#22756=CARTESIAN_POINT ( 'NONE',  ( -55.00000000000000000, 0.000000000000000000, 70.00000000000000000 ) ) ;
#22763=VECTOR ( 'NONE', #21620, 1000.000000000000000 ) ;
#22782=ORIENTED_EDGE ( 'NONE', *, *, #22646, .T. ) ;
#22786=VERTEX_POINT ( 'NONE', #14276 ) ;
#22804=ORIENTED_EDGE ( 'NONE', *, *, #8997, .T. ) ;
#22824=DIRECTION ( 'NONE',  ( 0.000000000000000000, 0.000000000000000000, -1.000000000000000000 ) ) ;
#22829=CIRCLE ( 'NONE', #16509, 11.00000000000001066 ) ;
#22838=ORIENTED_EDGE ( 'NONE', *, *, #3592, .F. ) ;
#22853=ORIENTED_EDGE ( 'NONE', *, *, #9976, .T. ) ;
#22864=CYLINDRICAL_SURFACE ( 'NONE', #31445, 11.00000000000000000 ) ;
#22906=DIRECTION ( 'NONE',  ( 0.000000000000000000, 0.000000000000000000, -1.000000000000000000 ) ) ;
#22915=CARTESIAN_POINT ( 'NONE',  ( 55.00000000000000000, 10.00000000000000888, 110.0000000000000000 ) ) ;
#22926=DIRECTION ( 'NONE',  ( 1.000000000000000000, -0.000000000000000000, -0.000000000000000000 ) ) ;
#22927=CARTESIAN_POINT ( 'NONE',  ( 46.00000000000000000, -25.98076211353320275, 73.99999999999992895 ) ) ;
#22982=CARTESIAN_POINT ( 'NONE',  ( -46.00000000000000000, -25.98076211353320275, 84.99999999999992895 ) ) ;
#23000=CIRCLE ( 'NONE', #28750, 7.999999999999992895 ) ;
#23004=FACE_OUTER_BOUND ( 'NONE', #33790, .T. ) ;
#23012=ORIENTED_EDGE ( 'NONE', *, *, #15581, .T. ) ;
#23064=ORIENTED_EDGE ( 'NONE', *, *, #23395, .F. ) ;
#23067=PLANE ( 'NONE',  #15908 ) ;
#23074=ADVANCED_FACE ( 'NONE', ( #1145 ), #4215, .F. ) ;
#23099=EDGE_LOOP ( 'NONE', ( #11457, #14598 ) ) ;
#23118=CARTESIAN_POINT ( 'NONE',  ( 50.00000000000000000, -25.98076211353320275, 84.99999999999992895 ) ) ;
#23176=DIRECTION ( 'NONE',  ( 0.000000000000000000, 0.000000000000000000, 1.000000000000000000 ) ) ;
#23191=ORIENTED_EDGE ( 'NONE', *, *, #34578, .T. ) ;
#23196=ORIENTED_EDGE ( 'NONE', *, *, #29138, .F. ) ;
#23231=ORIENTED_EDGE ( 'NONE', *, *, #6659, .F. ) ;
#23235=EDGE_LOOP ( 'NONE', ( #33844, #17288, #25606, #22656 ) ) ;
#23265=ADVANCED_FACE ( 'NONE', ( #23939 ), #7373, .F. ) ;
#23279=DIRECTION ( 'NONE',  ( 0.000000000000000000, 0.000000000000000000, -1.000000000000000000 ) ) ;
#23319=ORIENTED_EDGE ( 'NONE', *, *, #3122, .T. ) ;
#23327=ORIENTED_EDGE ( 'NONE', *, *, #5817, .T. ) ;
#23351=DIRECTION ( 'NONE',  ( 1.000000000000000000, 0.000000000000000000, -0.000000000000000000 ) ) ;
#23379=VERTEX_POINT ( 'NONE', #23572 ) ;
#23384=DIRECTION ( 'NONE',  ( 1.000000000000000000, -0.000000000000000000, -0.000000000000000000 ) ) ;
#23395=EDGE_CURVE ( 'NONE', #14544, #26283, #20871, .T. ) ;
#23397=CARTESIAN_POINT ( 'NONE',  ( 55.00000000000000000, 20.00000000000001776, 110.0000000000000000 ) ) ;
#23407=ADVANCED_FACE ( 'NONE', ( #27177 ), #30405, .F. ) ;
#23409=DIRECTION ( 'NONE',  ( 0.000000000000000000, 0.000000000000000000, -1.000000000000000000 ) ) ;
#23429=AXIS2_PLACEMENT_3D ( 'NONE', #29483, #23899, #12913 ) ;
#23438=CIRCLE ( 'NONE', #35534, 6.000000000000005329 ) ;
#23442=VERTEX_POINT ( 'NONE', #13145 ) ;
#23452=CIRCLE ( 'NONE', #19892, 5.000000000000011546 ) ;
#23458=AXIS2_PLACEMENT_3D ( 'NONE', #4683, #13136, #24115 ) ;
#23473=FACE_OUTER_BOUND ( 'NONE', #10647, .T. ) ;
#23480=ORIENTED_EDGE ( 'NONE', *, *, #12177, .F. ) ;
#23505=DIRECTION ( 'NONE',  ( -0.000000000000000000, -0.000000000000000000, -1.000000000000000000 ) ) ;
#23543=DIRECTION ( 'NONE',  ( 0.000000000000000000, -1.000000000000000000, 0.000000000000000000 ) ) ;
#23549=EDGE_CURVE ( 'NONE', #2539, #5260, #5035, .T. ) ;
#23556=EDGE_LOOP ( 'NONE', ( #30446, #22161 ) ) ;
#23572=CARTESIAN_POINT ( 'NONE',  ( -46.00000000000000000, -25.98076211353320275, 92.99999999999991473 ) ) ;
#23577=EDGE_CURVE ( 'NONE', #31687, #26586, #35281, .T. ) ;
#23607=ORIENTED_EDGE ( 'NONE', *, *, #28577, .F. ) ;
#23616=VECTOR ( 'NONE', #23505, 1000.000000000000000 ) ;
#23617=COLOUR_RGB ( '', 0.09019608, 0.27058824, 0.51372549) ;
#23621=CARTESIAN_POINT ( 'NONE',  ( 50.00000000000000000, 20.00000000000001776, -15.00000000000001421 ) ) ;
#23648=EDGE_CURVE ( 'NONE', #4839, #12825, #3216, .T. ) ;
#23678=CARTESIAN_POINT ( 'NONE',  ( 0.000000000000000000, 0.000000000000000000, 120.0000000000000000 ) ) ;
#23684=CARTESIAN_POINT ( 'NONE',  ( -50.00000000000000000, 10.00000000000000888, -25.00000000000000000 ) ) ;
#23693=EDGE_LOOP ( 'NONE', ( #24509, #28305, #34972, #13087 ) ) ;
#23710=CARTESIAN_POINT ( 'NONE',  ( -50.00000000000000000, 19.99999999999998934, -15.00000000000001421 ) ) ;
#23715=DIRECTION ( 'NONE',  ( -1.000000000000000000, -0.000000000000000000, -0.000000000000000000 ) ) ;
#23755=EDGE_LOOP ( 'NONE', ( #24193, #21929 ) ) ;
#23774=EDGE_CURVE ( 'NONE', #1635, #32416, #175, .T. ) ;
#23792=AXIS2_PLACEMENT_3D ( 'NONE', #26675, #16365, #27380 ) ;
#23816=DIRECTION ( 'NONE',  ( 0.000000000000000000, 0.000000000000000000, -1.000000000000000000 ) ) ;
#23838=CYLINDRICAL_SURFACE ( 'NONE', #19251, 10.00000000000000000 ) ;
#23840=EDGE_LOOP ( 'NONE', ( #24772, #30083 ) ) ;
#23844=DIRECTION ( 'NONE',  ( -1.000000000000000000, -0.000000000000000000, 0.000000000000000000 ) ) ;
#23860=DIRECTION ( 'NONE',  ( -1.000000000000000000, -1.387778780781445922E-16, 0.000000000000000000 ) ) ;
#23864=ORIENTED_EDGE ( 'NONE', *, *, #2000, .T. ) ;
#23870=DIRECTION ( 'NONE',  ( -0.000000000000000000, -0.000000000000000000, -1.000000000000000000 ) ) ;
#23899=DIRECTION ( 'NONE',  ( -1.000000000000000000, 0.000000000000000000, 0.000000000000000000 ) ) ;
#23923=CYLINDRICAL_SURFACE ( 'NONE', #1398, 11.00000000000000000 ) ;
#23939=FACE_OUTER_BOUND ( 'NONE', #16255, .T. ) ;
#23988=ORIENTED_EDGE ( 'NONE', *, *, #3122, .F. ) ;
#24001=CARTESIAN_POINT ( 'NONE',  ( -49.99999999999999289, -27.99999999999999289, 113.9999999999999858 ) ) ;
#24048=DIRECTION ( 'NONE',  ( 0.000000000000000000, 0.000000000000000000, -1.000000000000000000 ) ) ;
#24067=ORIENTED_EDGE ( 'NONE', *, *, #5044, .T. ) ;
#24073=ORIENTED_EDGE ( 'NONE', *, *, #33806, .T. ) ;
#24101=( NAMED_UNIT ( * ) PLANE_ANGLE_UNIT ( ) SI_UNIT ( $, .RADIAN. ) );
#24114=DIRECTION ( 'NONE',  ( 1.000000000000000000, -0.000000000000000000, -0.000000000000000000 ) ) ;
#24115=DIRECTION ( 'NONE',  ( 0.000000000000000000, 1.000000000000000000, 0.000000000000000000 ) ) ;
#24144=EDGE_LOOP ( 'NONE', ( #2470, #27330 ) ) ;
#24158=CIRCLE ( 'NONE', #29349, 10.00000000000000000 ) ;
#24193=ORIENTED_EDGE ( 'NONE', *, *, #18304, .T. ) ;
#24229=ADVANCED_FACE ( 'NONE', ( #6187, #28151 ), #11230, .F. ) ;
#24234=CARTESIAN_POINT ( 'NONE',  ( 46.00000000000000000, 0.000000000000000000, 70.00000000000000000 ) ) ;
#24249=CARTESIAN_POINT ( 'NONE',  ( -46.00000000000000000, -25.98076211353320275, 76.99999999999992895 ) ) ;
#24250=VERTEX_POINT ( 'NONE', #14813 ) ;
#24270=SURFACE_STYLE_USAGE ( .BOTH. , #29666 ) ;
#24280=CARTESIAN_POINT ( 'NONE',  ( 46.00000000000000000, 0.000000000000000000, 70.00000000000000000 ) ) ;
#24282=VERTEX_POINT ( 'NONE', #9594 ) ;
#24321=ORIENTED_EDGE ( 'NONE', *, *, #15804, .F. ) ;
#24329=LINE ( 'NONE', #13520, #10790 ) ;
#24340=ORIENTED_EDGE ( 'NONE', *, *, #11216, .F. ) ;
#24391=ADVANCED_FACE ( 'NONE', ( #9060 ), #4212, .F. ) ;
#24403=CARTESIAN_POINT ( 'NONE',  ( 46.00000000000000000, 0.000000000000000000, 70.00000000000000000 ) ) ;
#24422=EDGE_CURVE ( 'NONE', #15120, #29062, #7752, .T. ) ;
#24440=DIRECTION ( 'NONE',  ( 0.000000000000000000, -1.000000000000000000, 0.000000000000000000 ) ) ;
#24460=CYLINDRICAL_SURFACE ( 'NONE', #12724, 6.000000000000005329 ) ;
#24477=DIRECTION ( 'NONE',  ( -1.000000000000000000, -0.000000000000000000, -0.000000000000000000 ) ) ;
#24480=ADVANCED_FACE ( 'NONE', ( #2399 ), #2041, .T. ) ;
#24502=DIRECTION ( 'NONE',  ( 1.000000000000000000, -0.000000000000000000, 0.000000000000000000 ) ) ;
#24504=EDGE_CURVE ( 'NONE', #23442, #11697, #32444, .T. ) ;
#24505=VERTEX_POINT ( 'NONE', #21273 ) ;
#24509=ORIENTED_EDGE ( 'NONE', *, *, #12300, .F. ) ;
#24536=ORIENTED_EDGE ( 'NONE', *, *, #11054, .T. ) ;
#24550=VECTOR ( 'NONE', #19701, 1000.000000000000000 ) ;
#24591=EDGE_CURVE ( 'NONE', #22745, #12825, #18104, .T. ) ;
#24603=CARTESIAN_POINT ( 'NONE',  ( 46.00000000000000000, -25.98076211353320275, 76.99999999999992895 ) ) ;
#24614=DIRECTION ( 'NONE',  ( 1.000000000000000000, -0.000000000000000000, -0.000000000000000000 ) ) ;
#24633=CARTESIAN_POINT ( 'NONE',  ( -46.00000000000000000, 0.000000000000000000, 0.000000000000000000 ) ) ;
#24648=EDGE_LOOP ( 'NONE', ( #19622, #9024, #7960, #12353 ) ) ;
#24649=CARTESIAN_POINT ( 'NONE',  ( 0.000000000000000000, 10.00000000000000888, -15.00000000000000178 ) ) ;
#24686=ORIENTED_EDGE ( 'NONE', *, *, #13047, .T. ) ;
#24691=ORIENTED_EDGE ( 'NONE', *, *, #18679, .F. ) ;
#24721=AXIS2_PLACEMENT_3D ( 'NONE', #24649, #22622, #27708 ) ;
#24752=DIRECTION ( 'NONE',  ( -1.000000000000000000, -1.734723475976807094E-16, 0.000000000000000000 ) ) ;
#24759=CARTESIAN_POINT ( 'NONE',  ( -46.00000000000000000, -25.98076211353320275, 95.99999999999991473 ) ) ;
#24772=ORIENTED_EDGE ( 'NONE', *, *, #15804, .T. ) ;
#24842=DIRECTION ( 'NONE',  ( 1.734723475976807094E-16, -1.000000000000000000, 0.000000000000000000 ) ) ;
#24885=AXIS2_PLACEMENT_3D ( 'NONE', #12121, #20370, #6891 ) ;
#24916=EDGE_CURVE ( 'NONE', #22786, #3877, #26485, .T. ) ;
#24932=DIRECTION ( 'NONE',  ( 0.000000000000000000, 0.000000000000000000, -1.000000000000000000 ) ) ;
#24949=EDGE_LOOP ( 'NONE', ( #21027, #16464, #15751, #31048 ) ) ;
#24957=PLANE ( 'NONE',  #566 ) ;
#24996=VERTEX_POINT ( 'NONE', #12969 ) ;
#25020=CARTESIAN_POINT ( 'NONE',  ( -46.00000000000000000, 1.347111479062088405E-15, -11.00000000000000000 ) ) ;
#25028=CARTESIAN_POINT ( 'NONE',  ( -55.00000000000000000, -2.775557561562891351E-14, 110.0000000000000000 ) ) ;
#25033=DIRECTION ( 'NONE',  ( -1.000000000000000000, -1.734723475976807094E-16, -0.000000000000000000 ) ) ;
#25047=CIRCLE ( 'NONE', #7794, 8.000000000000007105 ) ;
#25067=ORIENTED_EDGE ( 'NONE', *, *, #8476, .T. ) ;
#25071=AXIS2_PLACEMENT_3D ( 'NONE', #14287, #977, #33919 ) ;
#25132=DIRECTION ( 'NONE',  ( -0.000000000000000000, 0.000000000000000000, -1.000000000000000000 ) ) ;
#25159=ORIENTED_EDGE ( 'NONE', *, *, #34052, .T. ) ;
#25162=CARTESIAN_POINT ( 'NONE',  ( 50.00000000000000000, 0.000000000000000000, 0.000000000000000000 ) ) ;
#25209=CIRCLE ( 'NONE', #3934, 8.000000000000012434 ) ;
#25216=DIRECTION ( 'NONE',  ( 0.000000000000000000, 0.000000000000000000, 1.000000000000000000 ) ) ;
#25282=LINE ( 'NONE', #970, #32632 ) ;
#25288=VECTOR ( 'NONE', #1800, 1000.000000000000000 ) ;
#25297=EDGE_LOOP ( 'NONE', ( #21917, #25159 ) ) ;
#25307=FACE_BOUND ( 'NONE', #10198, .T. ) ;
#25322=CARTESIAN_POINT ( 'NONE',  ( -46.00000000000000000, 0.000000000000000000, 81.00000000000001421 ) ) ;
#25334=CARTESIAN_POINT ( 'NONE',  ( -46.00000000000000000, 0.000000000000000000, 0.000000000000000000 ) ) ;
#25337=CIRCLE ( 'NONE', #38, 7.999999999999992895 ) ;
#25341=EDGE_LOOP ( 'NONE', ( #6776, #33872 ) ) ;
#25348=CARTESIAN_POINT ( 'NONE',  ( -46.00000000000000000, 0.000000000000000000, 0.000000000000000000 ) ) ;
#25356=ORIENTED_EDGE ( 'NONE', *, *, #1871, .F. ) ;
#25383=CARTESIAN_POINT ( 'NONE',  ( 46.00000000000000000, 0.000000000000000000, 61.99999999999999289 ) ) ;
#25418=VECTOR ( 'NONE', #16861, 1000.000000000000000 ) ;
#25442=AXIS2_PLACEMENT_3D ( 'NONE', #17519, #28522, #1330 ) ;
#25470=DIRECTION ( 'NONE',  ( 0.000000000000000000, 0.000000000000000000, 1.000000000000000000 ) ) ;
#25475=ORIENTED_EDGE ( 'NONE', *, *, #15461, .F. ) ;
#25492=DIRECTION ( 'NONE',  ( -1.000000000000000000, -0.000000000000000000, -0.000000000000000000 ) ) ;
#25534=CARTESIAN_POINT ( 'NONE',  ( 54.99999999999999289, -64.99999999999997158, -25.00000000000000000 ) ) ;
#25561=CIRCLE ( 'NONE', #4857, 10.99999999999999645 ) ;
#25589=AXIS2_PLACEMENT_3D ( 'NONE', #33973, #25877, #14868 ) ;
#25606=ORIENTED_EDGE ( 'NONE', *, *, #17908, .T. ) ;
#25622=ORIENTED_EDGE ( 'NONE', *, *, #18304, .F. ) ;
#25634=DIRECTION ( 'NONE',  ( 0.000000000000000000, 0.000000000000000000, -1.000000000000000000 ) ) ;
#25647=ORIENTED_EDGE ( 'NONE', *, *, #20666, .F. ) ;
#25652=ORIENTED_EDGE ( 'NONE', *, *, #7701, .F. ) ;
#25668=CIRCLE ( 'NONE', #17595, 4.000000000000003553 ) ;
#25678=AXIS2_PLACEMENT_3D ( 'NONE', #19292, #30302, #14070 ) ;
#25702=CIRCLE ( 'NONE', #22237, 10.00000000000000000 ) ;
#25703=LINE ( 'NONE', #12187, #18693 ) ;
#25745=CIRCLE ( 'NONE', #10216, 8.000000000000000000 ) ;
#25747=DIRECTION ( 'NONE',  ( 0.000000000000000000, 0.000000000000000000, -1.000000000000000000 ) ) ;
#25751=CYLINDRICAL_SURFACE ( 'NONE', #9267, 10.99999999999999645 ) ;
#25753=ORIENTED_EDGE ( 'NONE', *, *, #12804, .T. ) ;
#25758=VECTOR ( 'NONE', #19339, 1000.000000000000000 ) ;
#25796=ORIENTED_EDGE ( 'NONE', *, *, #33326, .F. ) ;
#25802=DIRECTION ( 'NONE',  ( 0.000000000000000000, 0.000000000000000000, 1.000000000000000000 ) ) ;
#25823=VERTEX_POINT ( 'NONE', #3901 ) ;
#25826=PLANE ( 'NONE',  #17083 ) ;
#25854=LINE ( 'NONE', #1899, #9943 ) ;
#25869=CARTESIAN_POINT ( 'NONE',  ( -50.00000000000000000, 0.000000000000000000, 0.000000000000000000 ) ) ;
#25874=DIRECTION ( 'NONE',  ( 0.000000000000000000, 1.000000000000000000, 0.000000000000000000 ) ) ;
#25876=ORIENTED_EDGE ( 'NONE', *, *, #9449, .T. ) ;
#25877=DIRECTION ( 'NONE',  ( 1.000000000000000000, 0.000000000000000000, 0.000000000000000000 ) ) ;
#25886=SHAPE_DEFINITION_REPRESENTATION ( #7225, #13971 ) ;
#25922=AXIS2_PLACEMENT_3D ( 'NONE', #6086, #22625, #23176 ) ;
#25924=DIRECTION ( 'NONE',  ( 1.000000000000000000, -0.000000000000000000, -0.000000000000000000 ) ) ;
#25965=CARTESIAN_POINT ( 'NONE',  ( -46.00000000000000000, 1.347111479062090574E-15, 59.00000000000000000 ) ) ;
#25970=DIRECTION ( 'NONE',  ( -1.000000000000000000, 0.000000000000000000, 0.000000000000000000 ) ) ;
#25997=EDGE_CURVE ( 'NONE', #19518, #26450, #28908, .T. ) ;
#26053=VECTOR ( 'NONE', #15101, 1000.000000000000000 ) ;
#26060=ORIENTED_EDGE ( 'NONE', *, *, #15180, .F. ) ;
#26064=DIRECTION ( 'NONE',  ( 0.000000000000000000, 0.000000000000000000, 1.000000000000000000 ) ) ;
#26088=EDGE_CURVE ( 'NONE', #29062, #1635, #4620, .T. ) ;
#26140=CARTESIAN_POINT ( 'NONE',  ( -55.00000000000000000, 6.123233995736780087E-16, 5.000000000000011546 ) ) ;
#26171=ORIENTED_EDGE ( 'NONE', *, *, #26827, .F. ) ;
#26200=DIRECTION ( 'NONE',  ( -1.000000000000000000, 0.000000000000000000, -0.000000000000000000 ) ) ;
#26206=FACE_OUTER_BOUND ( 'NONE', #32447, .T. ) ;
#26212=CARTESIAN_POINT ( 'NONE',  ( -46.00000000000000000, -25.98076211353320275, 84.99999999999992895 ) ) ;
#26225=CARTESIAN_POINT ( 'NONE',  ( 50.00000000000000000, 10.00000000000000888, 110.0000000000000000 ) ) ;
#26230=CARTESIAN_POINT ( 'NONE',  ( 50.00000000000000711, -25.98076211353320275, 78.99999999999992895 ) ) ;
#26232=ORIENTED_EDGE ( 'NONE', *, *, #32745, .F. ) ;
#26237=DIRECTION ( 'NONE',  ( -1.000000000000000000, -0.000000000000000000, -0.000000000000000000 ) ) ;
#26255=ORIENTED_EDGE ( 'NONE', *, *, #14093, .F. ) ;
#26262=VERTEX_POINT ( 'NONE', #11418 ) ;
#26265=CARTESIAN_POINT ( 'NONE',  ( 46.00000000000000000, -25.98076211353320275, 84.99999999999992895 ) ) ;
#26283=VERTEX_POINT ( 'NONE', #22556 ) ;
#26296=DIRECTION ( 'NONE',  ( 0.000000000000000000, 0.000000000000000000, -1.000000000000000000 ) ) ;
#26320=FACE_BOUND ( 'NONE', #4598, .T. ) ;
#26324=CARTESIAN_POINT ( 'NONE',  ( -50.00000000000000000, 10.00000000000000888, 110.0000000000000000 ) ) ;
#26354=LINE ( 'NONE', #35003, #21306 ) ;
#26363=VERTEX_POINT ( 'NONE', #19506 ) ;
#26368=ORIENTED_EDGE ( 'NONE', *, *, #7109, .F. ) ;
#26385=FACE_OUTER_BOUND ( 'NONE', #10913, .T. ) ;
#26392=PLANE ( 'NONE',  #3208 ) ;
#26418=DIRECTION ( 'NONE',  ( 1.000000000000000000, -0.000000000000000000, -0.000000000000000000 ) ) ;
#26425=CIRCLE ( 'NONE', #28732, 8.000000000000000000 ) ;
#26427=CARTESIAN_POINT ( 'NONE',  ( -50.00000000000000000, 0.000000000000000000, 70.00000000000000000 ) ) ;
#26438=FACE_OUTER_BOUND ( 'NONE', #31527, .T. ) ;
#26442=DIRECTION ( 'NONE',  ( -1.000000000000000000, -0.000000000000000000, -0.000000000000000000 ) ) ;
#26450=VERTEX_POINT ( 'NONE', #6534 ) ;
#26459=DIRECTION ( 'NONE',  ( 0.000000000000000000, 0.000000000000000000, -1.000000000000000000 ) ) ;
#26463=DIRECTION ( 'NONE',  ( 0.000000000000000000, 0.000000000000000000, -1.000000000000000000 ) ) ;
#26467=CARTESIAN_POINT ( 'NONE',  ( 46.00000000000000000, -25.98076211353320275, 76.99999999999992895 ) ) ;
#26485=LINE ( 'NONE', #4535, #16400 ) ;
#26494=ORIENTED_EDGE ( 'NONE', *, *, #17647, .F. ) ;
#26534=DIRECTION ( 'NONE',  ( 1.000000000000000000, -0.000000000000000000, -0.000000000000000000 ) ) ;
#26538=CARTESIAN_POINT ( 'NONE',  ( 55.00000000000000000, 10.00000000000000888, -25.00000000000000000 ) ) ;
#26571=VERTEX_POINT ( 'NONE', #34588 ) ;
#26586=VERTEX_POINT ( 'NONE', #31870 ) ;
#26589=CARTESIAN_POINT ( 'NONE',  ( 0.000000000000000000, 0.000000000000000000, 0.000000000000000000 ) ) ;
#26667=ORIENTED_EDGE ( 'NONE', *, *, #15610, .T. ) ;
#26674=ADVANCED_FACE ( 'NONE', ( #16359, #19241, #525, #16548, #13508, #13857 ), #8265, .F. ) ;
#26675=CARTESIAN_POINT ( 'NONE',  ( 50.00000000000000000, 20.00000000000001776, 120.0000000000000000 ) ) ;
#26758=DIRECTION ( 'NONE',  ( -1.000000000000000000, -0.000000000000000000, -0.000000000000000000 ) ) ;
#26783=CARTESIAN_POINT ( 'NONE',  ( 50.00000000000000711, -2.775557561562891351E-14, 110.0000000000000000 ) ) ;
#26793=CARTESIAN_POINT ( 'NONE',  ( -50.00000000000000000, 0.000000000000000000, 81.00000000000001421 ) ) ;
#26801=VERTEX_POINT ( 'NONE', #17070 ) ;
#26808=VECTOR ( 'NONE', #14109, 1000.000000000000000 ) ;
#26827=EDGE_CURVE ( 'NONE', #14470, #10703, #30251, .T. ) ;
#26913=EDGE_LOOP ( 'NONE', ( #18505, #19300 ) ) ;
#26942=CIRCLE ( 'NONE', #9080, 6.000000000000005329 ) ;
#26954=AXIS2_PLACEMENT_3D ( 'NONE', #25162, #33598, #12003 ) ;
#26966=EDGE_CURVE ( 'NONE', #6240, #26262, #29634, .T. ) ;
#26996=DIRECTION ( 'NONE',  ( 1.000000000000000000, 0.000000000000000000, 0.000000000000000000 ) ) ;
#27017=CARTESIAN_POINT ( 'NONE',  ( 55.00000000000000000, 20.00000000000001776, -25.00000000000000000 ) ) ;
#27020=ORIENTED_EDGE ( 'NONE', *, *, #31604, .T. ) ;
#27032=DIRECTION ( 'NONE',  ( 0.000000000000000000, 0.000000000000000000, -1.000000000000000000 ) ) ;
#27042=ORIENTED_EDGE ( 'NONE', *, *, #19802, .F. ) ;
#27070=DIRECTION ( 'NONE',  ( -0.000000000000000000, -1.000000000000000000, 0.000000000000000000 ) ) ;
#27108=FACE_OUTER_BOUND ( 'NONE', #18516, .T. ) ;
#27128=SURFACE_STYLE_FILL_AREA ( #16108 ) ;
#27177=FACE_OUTER_BOUND ( 'NONE', #15319, .T. ) ;
#27187=CARTESIAN_POINT ( 'NONE',  ( 46.00000000000000000, 0.000000000000000000, 0.000000000000000000 ) ) ;
#27239=ORIENTED_EDGE ( 'NONE', *, *, #23549, .F. ) ;
#27330=ORIENTED_EDGE ( 'NONE', *, *, #17864, .F. ) ;
#27333=DIRECTION ( 'NONE',  ( 0.000000000000000000, 0.000000000000000000, 1.000000000000000000 ) ) ;
#27380=DIRECTION ( 'NONE',  ( -0.000000000000000000, 0.000000000000000000, -1.000000000000000000 ) ) ;
#27397=CARTESIAN_POINT ( 'NONE',  ( -50.00000000000000000, 0.000000000000000000, 78.00000000000001421 ) ) ;
#27413=DIRECTION ( 'NONE',  ( -1.000000000000000000, -0.000000000000000000, 0.000000000000000000 ) ) ;
#27422=CIRCLE ( 'NONE', #9567, 10.99999999999999645 ) ;
#27428=AXIS2_PLACEMENT_3D ( 'NONE', #34497, #2627, #27470 ) ;
#27446=CARTESIAN_POINT ( 'NONE',  ( 50.00000000000000000, 0.000000000000000000, -8.000000000000000000 ) ) ;
#27470=DIRECTION ( 'NONE',  ( 0.000000000000000000, 0.000000000000000000, -1.000000000000000000 ) ) ;
#27484=( LENGTH_UNIT ( ) NAMED_UNIT ( * ) SI_UNIT ( .MILLI., .METRE. ) );
#27487=CIRCLE ( 'NONE', #11941, 11.00000000000000000 ) ;
#27488=FACE_OUTER_BOUND ( 'NONE', #28113, .T. ) ;
#27493=DIRECTION ( 'NONE',  ( 1.000000000000000000, 0.000000000000000000, -0.000000000000000000 ) ) ;
#27517=EDGE_LOOP ( 'NONE', ( #1919, #7735, #7143, #26368 ) ) ;
#27524=DIRECTION ( 'NONE',  ( 0.000000000000000000, 0.000000000000000000, 1.000000000000000000 ) ) ;
#27525=ADVANCED_FACE ( 'NONE', ( #17919 ), #15740, .F. ) ;
#27533=AXIS2_PLACEMENT_3D ( 'NONE', #20435, #6780, #17752 ) ;
#27534=DIRECTION ( 'NONE',  ( 1.000000000000000000, -0.000000000000000000, -0.000000000000000000 ) ) ;
#27546=CARTESIAN_POINT ( 'NONE',  ( -50.00000000000000000, 10.00000000000000888, -15.00000000000000178 ) ) ;
#27552=ORIENTED_EDGE ( 'NONE', *, *, #27641, .T. ) ;
#27568=DIRECTION ( 'NONE',  ( 0.000000000000000000, 0.000000000000000000, -1.000000000000000000 ) ) ;
#27573=EDGE_CURVE ( 'NONE', #2870, #30988, #2284, .T. ) ;
#27606=EDGE_CURVE ( 'NONE', #16063, #6941, #18814, .T. ) ;
#27639=DIRECTION ( 'NONE',  ( -1.000000000000000000, -1.387778780781445922E-16, -0.000000000000000000 ) ) ;
#27641=EDGE_CURVE ( 'NONE', #18294, #20350, #25047, .T. ) ;
#27708=DIRECTION ( 'NONE',  ( 0.000000000000000000, 0.000000000000000000, -1.000000000000000000 ) ) ;
#27721=ORIENTED_EDGE ( 'NONE', *, *, #13924, .F. ) ;
#27766=CARTESIAN_POINT ( 'NONE',  ( 46.00000000000000000, 0.000000000000000000, 0.000000000000000000 ) ) ;
#27774=CARTESIAN_POINT ( 'NONE',  ( 46.00000000000000000, -25.98076211353320275, 84.99999999999992895 ) ) ;
#27790=ORIENTED_EDGE ( 'NONE', *, *, #4310, .T. ) ;
#27808=ORIENTED_EDGE ( 'NONE', *, *, #24591, .F. ) ;
#27831=AXIS2_PLACEMENT_3D ( 'NONE', #19941, #30597, #27899 ) ;
#27835=ADVANCED_FACE ( 'NONE', ( #20203 ), #6196, .T. ) ;
#27854=DIRECTION ( 'NONE',  ( 0.000000000000000000, 0.000000000000000000, 1.000000000000000000 ) ) ;
#27856=ORIENTED_EDGE ( 'NONE', *, *, #25997, .F. ) ;
#27868=EDGE_CURVE ( 'NONE', #31582, #17845, #6538, .T. ) ;
#27884=AXIS2_PLACEMENT_3D ( 'NONE', #34262, #28689, #34453 ) ;
#27899=DIRECTION ( 'NONE',  ( 0.000000000000000000, 0.000000000000000000, 1.000000000000000000 ) ) ;
#27963=DIRECTION ( 'NONE',  ( 1.000000000000000000, 0.000000000000000000, 0.000000000000000000 ) ) ;
#27964=LINE ( 'NONE', #33537, #20527 ) ;
#27988=DIRECTION ( 'NONE',  ( -1.734723475976807094E-16, 1.000000000000000000, -0.000000000000000000 ) ) ;
#27994=ORIENTED_EDGE ( 'NONE', *, *, #13734, .F. ) ;
#28002=DIRECTION ( 'NONE',  ( 1.000000000000000000, -0.000000000000000000, -0.000000000000000000 ) ) ;
#28014=DIRECTION ( 'NONE',  ( 0.000000000000000000, 0.000000000000000000, 1.000000000000000000 ) ) ;
#28018=PLANE ( 'NONE',  #15126 ) ;
#28045=ORIENTED_EDGE ( 'NONE', *, *, #29391, .T. ) ;
#28059=DIRECTION ( 'NONE',  ( 0.000000000000000000, -1.000000000000000000, 0.000000000000000000 ) ) ;
#28094=CARTESIAN_POINT ( 'NONE',  ( -29.99999999999999645, -26.99999999999999645, 113.9999999999999858 ) ) ;
#28113=EDGE_LOOP ( 'NONE', ( #4096, #12005, #17113, #19052 ) ) ;
#28125=ORIENTED_EDGE ( 'NONE', *, *, #30015, .T. ) ;
#28135=ORIENTED_EDGE ( 'NONE', *, *, #32604, .T. ) ;
#28139=CARTESIAN_POINT ( 'NONE',  ( -55.00000000000000000, 0.000000000000000000, 0.000000000000000000 ) ) ;
#28140=COLOUR_RGB ( '', 0.09019608, 0.27058824, 0.51372549) ;
#28147=DIRECTION ( 'NONE',  ( -1.000000000000000000, -0.000000000000000000, 0.000000000000000000 ) ) ;
#28151=FACE_OUTER_BOUND ( 'NONE', #8964, .T. ) ;
#28156=CIRCLE ( 'NONE', #9755, 5.000000000000011546 ) ;
#28169=CARTESIAN_POINT ( 'NONE',  ( -46.00000000000000000, -25.98076211353320275, 84.99999999999992895 ) ) ;
#28175=EDGE_LOOP ( 'NONE', ( #29148, #24340, #6204, #5731 ) ) ;
#28190=ADVANCED_FACE ( 'NONE', ( #23004 ), #14896, .F. ) ;
#28213=DIRECTION ( 'NONE',  ( -1.000000000000000000, -1.734723475976807094E-16, 0.000000000000000000 ) ) ;
#28227=AXIS2_PLACEMENT_3D ( 'NONE', #26427, #23715, #15413 ) ;
#28267=DIRECTION ( 'NONE',  ( 0.000000000000000000, 0.000000000000000000, 1.000000000000000000 ) ) ;
#28277=DIRECTION ( 'NONE',  ( 0.000000000000000000, 0.000000000000000000, -1.000000000000000000 ) ) ;
#28278=DIRECTION ( 'NONE',  ( 0.000000000000000000, -1.000000000000000000, 0.000000000000000000 ) ) ;
#28305=ORIENTED_EDGE ( 'NONE', *, *, #34346, .F. ) ;
#28306=CARTESIAN_POINT ( 'NONE',  ( -49.99999999999998579, -60.00000000000000000, 120.0000000000000000 ) ) ;
#28320=CARTESIAN_POINT ( 'NONE',  ( -49.99999999999999289, -25.98076211353320275, 84.99999999999994316 ) ) ;
#28338=ORIENTED_EDGE ( 'NONE', *, *, #22742, .F. ) ;
#28340=DIRECTION ( 'NONE',  ( 0.000000000000000000, 0.000000000000000000, -1.000000000000000000 ) ) ;
#28349=VERTEX_POINT ( 'NONE', #26793 ) ;
#28360=DIRECTION ( 'NONE',  ( -1.000000000000000000, -1.734723475976807094E-16, 0.000000000000000000 ) ) ;
#28364=VERTEX_POINT ( 'NONE', #34718 ) ;
#28369=DIRECTION ( 'NONE',  ( 1.000000000000000000, -0.000000000000000000, -0.000000000000000000 ) ) ;
#28385=EDGE_LOOP ( 'NONE', ( #536, #12498 ) ) ;
#28397=ADVANCED_FACE ( 'NONE', ( #26438 ), #34539, .T. ) ;
#28403=CARTESIAN_POINT ( 'NONE',  ( 50.00000000000000000, -59.99999999999997158, 120.0000000000000000 ) ) ;
#28433=FACE_OUTER_BOUND ( 'NONE', #6541, .T. ) ;
#28439=ADVANCED_FACE ( 'NONE', ( #1769 ), #12573, .T. ) ;
#28471=DIRECTION ( 'NONE',  ( 1.000000000000000000, -0.000000000000000000, -0.000000000000000000 ) ) ;
#28484=ORIENTED_EDGE ( 'NONE', *, *, #3857, .T. ) ;
#28486=CARTESIAN_POINT ( 'NONE',  ( 50.00000000000000000, -25.98076211353320275, 84.99999999999992895 ) ) ;
#28509=DIRECTION ( 'NONE',  ( -1.000000000000000000, -1.734723475976807094E-16, 0.000000000000000000 ) ) ;
#28512=CARTESIAN_POINT ( 'NONE',  ( 50.00000000000000000, 20.00000000000001776, 120.0000000000000000 ) ) ;
#28522=DIRECTION ( 'NONE',  ( -1.000000000000000000, -0.000000000000000000, -0.000000000000000000 ) ) ;
#28530=ORIENTED_EDGE ( 'NONE', *, *, #11610, .F. ) ;
#28543=VECTOR ( 'NONE', #27988, 1000.000000000000000 ) ;
#28545=CYLINDRICAL_SURFACE ( 'NONE', #30705, 11.00000000000001066 ) ;
#28557=FACE_OUTER_BOUND ( 'NONE', #5892, .T. ) ;
#28565=EDGE_CURVE ( 'NONE', #16796, #6240, #5364, .T. ) ;
#28577=EDGE_CURVE ( 'NONE', #24996, #9078, #4985, .T. ) ;
#28580=VERTEX_POINT ( 'NONE', #16309 ) ;
#28585=CARTESIAN_POINT ( 'NONE',  ( 50.00000000000000711, 0.000000000000000000, 64.00000000000000000 ) ) ;
#28639=DIRECTION ( 'NONE',  ( 1.000000000000000000, -0.000000000000000000, -0.000000000000000000 ) ) ;
#28689=DIRECTION ( 'NONE',  ( -1.000000000000000000, -0.000000000000000000, -0.000000000000000000 ) ) ;
#28713=EDGE_LOOP ( 'NONE', ( #12413, #10151, #35206, #8313 ) ) ;
#28732=AXIS2_PLACEMENT_3D ( 'NONE', #15272, #31508, #21031 ) ;
#28738=DIRECTION ( 'NONE',  ( 0.000000000000000000, 0.000000000000000000, 1.000000000000000000 ) ) ;
#28750=AXIS2_PLACEMENT_3D ( 'NONE', #16171, #14014, #8437 ) ;
#28751=DIRECTION ( 'NONE',  ( 0.000000000000000000, 0.000000000000000000, 1.000000000000000000 ) ) ;
#28784=VERTEX_POINT ( 'NONE', #9110 ) ;
#28797=ORIENTED_EDGE ( 'NONE', *, *, #3592, .T. ) ;
#28802=CIRCLE ( 'NONE', #7517, 6.000000000000005329 ) ;
#28822=EDGE_CURVE ( 'NONE', #22338, #1992, #19924, .T. ) ;
#28834=FACE_BOUND ( 'NONE', #31868, .T. ) ;
#28877=ORIENTED_EDGE ( 'NONE', *, *, #7142, .T. ) ;
#28887=EDGE_CURVE ( 'NONE', #5884, #8628, #5015, .T. ) ;
#28899=VERTEX_POINT ( 'NONE', #23684 ) ;
#28905=DIRECTION ( 'NONE',  ( 0.000000000000000000, 0.000000000000000000, -1.000000000000000000 ) ) ;
#28908=LINE ( 'NONE', #2096, #18214 ) ;
#28916=EDGE_LOOP ( 'NONE', ( #10919, #21289, #25647, #19648 ) ) ;
#28927=FACE_OUTER_BOUND ( 'NONE', #3598, .T. ) ;
#28931=DIRECTION ( 'NONE',  ( 1.000000000000000000, -0.000000000000000000, 0.000000000000000000 ) ) ;
#28943=AXIS2_PLACEMENT_3D ( 'NONE', #5139, #32672, #24048 ) ;
#28949=LINE ( 'NONE', #5003, #10964 ) ;
#28977=CIRCLE ( 'NONE', #27831, 11.00000000000000000 ) ;
#28984=DIRECTION ( 'NONE',  ( 0.000000000000000000, -1.000000000000000000, 0.000000000000000000 ) ) ;
#29004=CARTESIAN_POINT ( 'NONE',  ( -55.00000000000000000, 0.000000000000000000, 0.000000000000000000 ) ) ;
#29009=ADVANCED_FACE ( 'NONE', ( #26206 ), #1544, .F. ) ;
#29011=ORIENTED_EDGE ( 'NONE', *, *, #35571, .F. ) ;
#29014=DIRECTION ( 'NONE',  ( 0.000000000000000000, -1.000000000000000000, 0.000000000000000000 ) ) ;
#29062=VERTEX_POINT ( 'NONE', #19508 ) ;
#29086=PLANE ( 'NONE',  #17065 ) ;
#29115=EDGE_CURVE ( 'NONE', #12825, #22745, #33196, .T. ) ;
#29138=EDGE_CURVE ( 'NONE', #32964, #35140, #25282, .T. ) ;
#29139=CARTESIAN_POINT ( 'NONE',  ( -46.00000000000000000, -25.98076211353320275, 84.99999999999992895 ) ) ;
#29140=CARTESIAN_POINT ( 'NONE',  ( -55.00000000000000000, 7.347880794884122694E-16, 76.00000000000001421 ) ) ;
#29148=ORIENTED_EDGE ( 'NONE', *, *, #30171, .F. ) ;
#29222=DIRECTION ( 'NONE',  ( 0.000000000000000000, 0.000000000000000000, -1.000000000000000000 ) ) ;
#29224=CIRCLE ( 'NONE', #33246, 10.99999999999999645 ) ;
#29249=VECTOR ( 'NONE', #21268, 1000.000000000000000 ) ;
#29262=EDGE_CURVE ( 'NONE', #30657, #2467, #17154, .T. ) ;
#29263=ADVANCED_FACE ( 'NONE', ( #3504, #11761 ), #25826, .F. ) ;
#29272=VECTOR ( 'NONE', #17847, 1000.000000000000000 ) ;
#29275=CARTESIAN_POINT ( 'NONE',  ( -50.00000000000000000, -2.775557561562891351E-14, 110.0000000000000000 ) ) ;
#29285=DIRECTION ( 'NONE',  ( -1.000000000000000000, -1.734723475976807094E-16, 0.000000000000000000 ) ) ;
#29335=CYLINDRICAL_SURFACE ( 'NONE', #30928, 11.00000000000001066 ) ;
#29349=AXIS2_PLACEMENT_3D ( 'NONE', #27546, #18890, #2533 ) ;
#29391=EDGE_CURVE ( 'NONE', #35140, #28899, #24329, .T. ) ;
#29404=ORIENTED_EDGE ( 'NONE', *, *, #24916, .T. ) ;
#29465=EDGE_LOOP ( 'NONE', ( #20440, #25753 ) ) ;
#29466=( LENGTH_UNIT ( ) NAMED_UNIT ( * ) SI_UNIT ( .MILLI., .METRE. ) );
#29472=ADVANCED_FACE ( 'NONE', ( #30258 ), #22654, .F. ) ;
#29483=CARTESIAN_POINT ( 'NONE',  ( 50.00000000000000000, 0.000000000000000000, 0.000000000000000000 ) ) ;
#29506=DIRECTION ( 'NONE',  ( 0.000000000000000000, 0.000000000000000000, 1.000000000000000000 ) ) ;
#29517=CARTESIAN_POINT ( 'NONE',  ( -55.00000000000000000, -2.775557561562891351E-14, 110.0000000000000000 ) ) ;
#29527=CARTESIAN_POINT ( 'NONE',  ( -55.00000000000000000, -25.98076211353320275, 84.99999999999994316 ) ) ;
#29531=VECTOR ( 'NONE', #24614, 1000.000000000000000 ) ;
#29584=DIRECTION ( 'NONE',  ( -1.734723475976807094E-16, 1.000000000000000000, -0.000000000000000000 ) ) ;
#29589=DIRECTION ( 'NONE',  ( 0.000000000000000000, -1.000000000000000000, 0.000000000000000000 ) ) ;
#29630=DIRECTION ( 'NONE',  ( 0.000000000000000000, -1.000000000000000000, 0.000000000000000000 ) ) ;
#29632=DIRECTION ( 'NONE',  ( 0.000000000000000000, 0.000000000000000000, 1.000000000000000000 ) ) ;
#29634=CIRCLE ( 'NONE', #33616, 10.99999999999999645 ) ;
#29659=CARTESIAN_POINT ( 'NONE',  ( 46.00000000000000000, 1.347111479062088405E-15, 11.00000000000000000 ) ) ;
#29664=ADVANCED_FACE ( 'NONE', ( #28433 ), #14735, .F. ) ;
#29666=SURFACE_SIDE_STYLE ('',( #1953 ) ) ;
#29709=AXIS2_PLACEMENT_3D ( 'NONE', #7478, #34864, #2285 ) ;
#29717=ADVANCED_FACE ( 'NONE', ( #12230 ), #20484, .T. ) ;
#29726=ORIENTED_EDGE ( 'NONE', *, *, #30015, .F. ) ;
#29737=CARTESIAN_POINT ( 'NONE',  ( -55.00000000000000000, 0.000000000000000000, 70.00000000000000000 ) ) ;
#29764=CIRCLE ( 'NONE', #23429, 8.000000000000000000 ) ;
#29801=ADVANCED_FACE ( 'NONE', ( #2338 ), #29335, .T. ) ;
#29825=ORIENTED_EDGE ( 'NONE', *, *, #32604, .F. ) ;
#29829=ORIENTED_EDGE ( 'NONE', *, *, #16524, .F. ) ;
#29869=DIRECTION ( 'NONE',  ( -1.000000000000000000, -0.000000000000000000, -0.000000000000000000 ) ) ;
#29885=CARTESIAN_POINT ( 'NONE',  ( -55.00000000000000000, -2.726571689596996976E-14, 114.0000000000000000 ) ) ;
#29903=PLANE ( 'NONE',  #23792 ) ;
#29942=DIRECTION ( 'NONE',  ( -1.000000000000000000, -0.000000000000000000, -0.000000000000000000 ) ) ;
#29969=AXIS2_PLACEMENT_3D ( 'NONE', #2941, #7780, #19287 ) ;
#29986=CARTESIAN_POINT ( 'NONE',  ( 50.00000000000000000, 0.000000000000000000, 70.00000000000000000 ) ) ;
#29992=EDGE_LOOP ( 'NONE', ( #8461, #24321, #28797, #33653 ) ) ;
#29996=EDGE_CURVE ( 'NONE', #16003, #2539, #20892, .T. ) ;
#30003=VECTOR ( 'NONE', #29869, 1000.000000000000000 ) ;
#30014=DIRECTION ( 'NONE',  ( -1.000000000000000000, -0.000000000000000000, -0.000000000000000000 ) ) ;
#30015=EDGE_CURVE ( 'NONE', #33645, #864, #22065, .T. ) ;
#30033=ADVANCED_FACE ( 'NONE', ( #22272 ), #21738, .T. ) ;
#30036=VERTEX_POINT ( 'NONE', #32732 ) ;
#30053=CARTESIAN_POINT ( 'NONE',  ( -46.00000000000000000, 0.000000000000000000, 81.00000000000001421 ) ) ;
#30060=CARTESIAN_POINT ( 'NONE',  ( 50.00000000000000000, 0.000000000000000000, 0.000000000000000000 ) ) ;
#30083=ORIENTED_EDGE ( 'NONE', *, *, #22742, .T. ) ;
#30121=ORIENTED_EDGE ( 'NONE', *, *, #30171, .T. ) ;
#30155=DIRECTION ( 'NONE',  ( 0.000000000000000000, 0.000000000000000000, -1.000000000000000000 ) ) ;
#30158=CARTESIAN_POINT ( 'NONE',  ( 50.00000000000000711, 6.123233995736780087E-16, 5.000000000000011546 ) ) ;
#30159=ADVANCED_FACE ( 'NONE', ( #4770 ), #23838, .T. ) ;
#30169=VERTEX_POINT ( 'NONE', #30916 ) ;
#30171=EDGE_CURVE ( 'NONE', #3309, #1992, #25703, .T. ) ;
#30214=DIRECTION ( 'NONE',  ( 0.000000000000000000, 0.000000000000000000, -1.000000000000000000 ) ) ;
#30218=CARTESIAN_POINT ( 'NONE',  ( 50.00000000000000000, 10.00000000000000888, 120.0000000000000000 ) ) ;
#30219=ORIENTED_EDGE ( 'NONE', *, *, #28565, .F. ) ;
#30240=VECTOR ( 'NONE', #12887, 1000.000000000000000 ) ;
#30251=CIRCLE ( 'NONE', #22661, 5.000000000000011546 ) ;
#30258=FACE_OUTER_BOUND ( 'NONE', #18563, .T. ) ;
#30263=CYLINDRICAL_SURFACE ( 'NONE', #21885, 0.9999999999999974465 ) ;
#30264=EDGE_LOOP ( 'NONE', ( #17151, #22702 ) ) ;
#30286=CARTESIAN_POINT ( 'NONE',  ( 50.00000000000000000, 0.000000000000000000, 70.00000000000000000 ) ) ;
#30297=PLANE ( 'NONE',  #19574 ) ;
#30302=DIRECTION ( 'NONE',  ( 1.000000000000000000, -0.000000000000000000, -0.000000000000000000 ) ) ;
#30352=ORIENTED_EDGE ( 'NONE', *, *, #12804, .F. ) ;
#30363=FACE_BOUND ( 'NONE', #9841, .T. ) ;
#30364=FACE_BOUND ( 'NONE', #17347, .T. ) ;
#30396=DIRECTION ( 'NONE',  ( 1.734723475976807094E-16, -1.000000000000000000, 0.000000000000000000 ) ) ;
#30405=CYLINDRICAL_SURFACE ( 'NONE', #20273, 5.000000000000011546 ) ;
#30421=CARTESIAN_POINT ( 'NONE',  ( -29.99999999999999645, -26.00000000000000000, 113.9999999999999858 ) ) ;
#30445=FACE_OUTER_BOUND ( 'NONE', #29992, .T. ) ;
#30446=ORIENTED_EDGE ( 'NONE', *, *, #31301, .T. ) ;
#30496=CARTESIAN_POINT ( 'NONE',  ( -55.00000000000000000, 0.000000000000000000, 70.00000000000000000 ) ) ;
#30503=EDGE_LOOP ( 'NONE', ( #17398, #24686, #26494, #21298 ) ) ;
#30514=DIRECTION ( 'NONE',  ( 1.000000000000000000, -0.000000000000000000, -0.000000000000000000 ) ) ;
#30529=STYLED_ITEM ( 'NONE', ( #10729 ), #12087 ) ;
#30546=ORIENTED_EDGE ( 'NONE', *, *, #10595, .F. ) ;
#30574=CYLINDRICAL_SURFACE ( 'NONE', #24721, 10.00000000000000000 ) ;
#30597=DIRECTION ( 'NONE',  ( -1.000000000000000000, 0.000000000000000000, 0.000000000000000000 ) ) ;
#30604=ORIENTED_EDGE ( 'NONE', *, *, #29996, .F. ) ;
#30610=FACE_OUTER_BOUND ( 'NONE', #15257, .T. ) ;
#30620=CARTESIAN_POINT ( 'NONE',  ( -55.00000000000000000, 10.00000000000000888, -15.00000000000000178 ) ) ;
#30634=VERTEX_POINT ( 'NONE', #23621 ) ;
#30657=VERTEX_POINT ( 'NONE', #26140 ) ;
#30688=EDGE_CURVE ( 'NONE', #21944, #24250, #4103, .T. ) ;
#30705=AXIS2_PLACEMENT_3D ( 'NONE', #31594, #25492, #17903 ) ;
#30723=DIRECTION ( 'NONE',  ( -1.000000000000000000, -0.000000000000000000, -0.000000000000000000 ) ) ;
#30740=ORIENTED_EDGE ( 'NONE', *, *, #12300, .T. ) ;
#30761=ORIENTED_EDGE ( 'NONE', *, *, #8476, .F. ) ;
#30779=CARTESIAN_POINT ( 'NONE',  ( -46.00000000000000000, 0.000000000000000000, 70.00000000000000000 ) ) ;
#30801=ORIENTED_EDGE ( 'NONE', *, *, #3829, .T. ) ;
#30841=ADVANCED_FACE ( 'NONE', ( #15668 ), #2385, .F. ) ;
#30908=DIRECTION ( 'NONE',  ( 0.000000000000000000, 0.000000000000000000, 1.000000000000000000 ) ) ;
#30916=CARTESIAN_POINT ( 'NONE',  ( 50.00000000000000000, -25.98076211353320275, 92.99999999999991473 ) ) ;
#30928=AXIS2_PLACEMENT_3D ( 'NONE', #10053, #24114, #12764 ) ;
#30988=VERTEX_POINT ( 'NONE', #33312 ) ;
#30995=ADVANCED_FACE ( 'NONE', ( #30445 ), #30263, .T. ) ;
#30999=ADVANCED_FACE ( 'NONE', ( #30610, #2911 ), #3254, .T. ) ;
#31048=ORIENTED_EDGE ( 'NONE', *, *, #33286, .F. ) ;
#31052=AXIS2_PLACEMENT_3D ( 'NONE', #30496, #27963, #33363 ) ;
#31059=CARTESIAN_POINT ( 'NONE',  ( 46.00000000000000000, 9.797174393178841435E-16, 78.00000000000001421 ) ) ;
#31061=VECTOR ( 'NONE', #34333, 1000.000000000000000 ) ;
#31086=CARTESIAN_POINT ( 'NONE',  ( -50.00000000000000000, 0.000000000000000000, 70.00000000000000000 ) ) ;
#31104=ORIENTED_EDGE ( 'NONE', *, *, #4310, .F. ) ;
#31116=ADVANCED_FACE ( 'NONE', ( #9527 ), #25751, .T. ) ;
#31140=CIRCLE ( 'NONE', #4721, 8.000000000000000000 ) ;
#31142=ORIENTED_EDGE ( 'NONE', *, *, #31543, .F. ) ;
#31154=DIRECTION ( 'NONE',  ( -1.000000000000000000, -0.000000000000000000, -0.000000000000000000 ) ) ;
#31237=CARTESIAN_POINT ( 'NONE',  ( 46.00000000000000000, 0.000000000000000000, 61.99999999999999289 ) ) ;
#31248=CARTESIAN_POINT ( 'NONE',  ( -46.00000000000000000, -25.98076211353320275, 76.99999999999992895 ) ) ;
#31258=DIRECTION ( 'NONE',  ( 0.000000000000000000, -0.000000000000000000, 1.000000000000000000 ) ) ;
#31299=CARTESIAN_POINT ( 'NONE',  ( 50.00000000000000711, 0.000000000000000000, 0.000000000000000000 ) ) ;
#31301=EDGE_CURVE ( 'NONE', #17702, #33466, #1803, .T. ) ;
#31307=ORIENTED_EDGE ( 'NONE', *, *, #31604, .F. ) ;
#31311=ORIENTED_EDGE ( 'NONE', *, *, #12761, .F. ) ;
#31314=EDGE_CURVE ( 'NONE', #25823, #24996, #1794, .T. ) ;
#31326=DIRECTION ( 'NONE',  ( -1.000000000000000000, -1.734723475976807094E-16, 0.000000000000000000 ) ) ;
#31346=EDGE_LOOP ( 'NONE', ( #35540, #20915, #16148, #13225 ) ) ;
#31381=DIRECTION ( 'NONE',  ( 0.000000000000000000, 0.000000000000000000, -1.000000000000000000 ) ) ;
#31397=ORIENTED_EDGE ( 'NONE', *, *, #7741, .F. ) ;
#31414=VECTOR ( 'NONE', #33414, 1000.000000000000000 ) ;
#31429=CARTESIAN_POINT ( 'NONE',  ( -50.00000000000000000, -2.775557561562891351E-14, 106.0000000000000000 ) ) ;
#31445=AXIS2_PLACEMENT_3D ( 'NONE', #33860, #31154, #20148 ) ;
#31460=ADVANCED_FACE ( 'NONE', ( #13478 ), #24460, .F. ) ;
#31508=DIRECTION ( 'NONE',  ( -1.000000000000000000, 0.000000000000000000, 0.000000000000000000 ) ) ;
#31527=EDGE_LOOP ( 'NONE', ( #30219, #9160, #23864, #19562 ) ) ;
#31543=EDGE_CURVE ( 'NONE', #3309, #7646, #31140, .T. ) ;
#31545=EDGE_CURVE ( 'NONE', #22786, #11158, #661, .T. ) ;
#31582=VERTEX_POINT ( 'NONE', #30218 ) ;
#31594=CARTESIAN_POINT ( 'NONE',  ( -46.00000000000000000, 0.000000000000000000, 70.00000000000000000 ) ) ;
#31604=EDGE_CURVE ( 'NONE', #23379, #31888, #11600, .T. ) ;
#31622=CARTESIAN_POINT ( 'NONE',  ( 50.00000000000000000, 9.797174393178845379E-16, 78.00000000000001421 ) ) ;
#31630=LINE ( 'NONE', #4288, #33195 ) ;
#31667=DIRECTION ( 'NONE',  ( 1.000000000000000000, -0.000000000000000000, -0.000000000000000000 ) ) ;
#31687=VERTEX_POINT ( 'NONE', #26230 ) ;
#31706=CARTESIAN_POINT ( 'NONE',  ( -55.00000000000000000, 19.99999999999998934, 120.0000000000000000 ) ) ;
#31736=LINE ( 'NONE', #9951, #3646 ) ;
#31737=EDGE_LOOP ( 'NONE', ( #30761, #12815, #17790, #27994 ) ) ;
#31821=AXIS2_PLACEMENT_3D ( 'NONE', #27766, #3106, #14410 ) ;
#31824=FILL_AREA_STYLE_COLOUR ( '', #28140 ) ;
#31863=ORIENTED_EDGE ( 'NONE', *, *, #22056, .F. ) ;
#31866=ORIENTED_EDGE ( 'NONE', *, *, #33847, .T. ) ;
#31868=EDGE_LOOP ( 'NONE', ( #4808, #35589 ) ) ;
#31870=CARTESIAN_POINT ( 'NONE',  ( 50.00000000000000711, -25.98076211353320275, 90.99999999999994316 ) ) ;
#31885=DIRECTION ( 'NONE',  ( -1.000000000000000000, -0.000000000000000000, -0.000000000000000000 ) ) ;
#31888=VERTEX_POINT ( 'NONE', #24249 ) ;
#31899=DIRECTION ( 'NONE',  ( -1.000000000000000000, -0.000000000000000000, -0.000000000000000000 ) ) ;
#31958=DIRECTION ( 'NONE',  ( -1.000000000000000000, 0.000000000000000000, -0.000000000000000000 ) ) ;
#31974=EDGE_LOOP ( 'NONE', ( #7846, #31307, #2057, #9729 ) ) ;
#31992=EDGE_LOOP ( 'NONE', ( #23480, #15828, #24536, #20966 ) ) ;
#32020=DIRECTION ( 'NONE',  ( 0.000000000000000000, 0.000000000000000000, 1.000000000000000000 ) ) ;
#32021=CARTESIAN_POINT ( 'NONE',  ( -50.00000000000000000, 9.797174393178825657E-16, -8.000000000000000000 ) ) ;
#32025=VERTEX_POINT ( 'NONE', #33234 ) ;
#32031=VECTOR ( 'NONE', #34900, 1000.000000000000000 ) ;
#32054=CARTESIAN_POINT ( 'NONE',  ( -55.00000000000000000, -25.98076211353320275, 90.99999999999994316 ) ) ;
#32075=DIRECTION ( 'NONE',  ( 0.000000000000000000, 0.000000000000000000, 1.000000000000000000 ) ) ;
#32081=ORIENTED_EDGE ( 'NONE', *, *, #8594, .T. ) ;
#32154=CARTESIAN_POINT ( 'NONE',  ( 50.00000000000000711, -2.726571689596996976E-14, 114.0000000000000000 ) ) ;
#32164=AXIS2_PLACEMENT_3D ( 'NONE', #34887, #21709, #2836 ) ;
#32198=DIRECTION ( 'NONE',  ( 0.000000000000000000, 0.000000000000000000, -1.000000000000000000 ) ) ;
#32224=DIRECTION ( 'NONE',  ( -1.000000000000000000, 0.000000000000000000, 0.000000000000000000 ) ) ;
#32230=ORIENTED_EDGE ( 'NONE', *, *, #28822, .F. ) ;
#32262=DIRECTION ( 'NONE',  ( 0.000000000000000000, 0.000000000000000000, 1.000000000000000000 ) ) ;
#32271=CARTESIAN_POINT ( 'NONE',  ( 55.00000000000000000, -2.775557561562891351E-14, 110.0000000000000000 ) ) ;
#32333=FILL_AREA_STYLE_COLOUR ( '', #23617 ) ;
#32409=ORIENTED_EDGE ( 'NONE', *, *, #3857, .F. ) ;
#32416=VERTEX_POINT ( 'NONE', #16070 ) ;
#32425=EDGE_LOOP ( 'NONE', ( #22541, #22092, #17939, #34347 ) ) ;
#32443=LINE ( 'NONE', #18752, #22763 ) ;
#32444=LINE ( 'NONE', #10486, #16936 ) ;
#32447=EDGE_LOOP ( 'NONE', ( #10112, #33098, #12401, #21580 ) ) ;
#32473=DIRECTION ( 'NONE',  ( 0.000000000000000000, 0.000000000000000000, -1.000000000000000000 ) ) ;
#32504=SURFACE_SIDE_STYLE ('',( #27128 ) ) ;
#32561=FACE_OUTER_BOUND ( 'NONE', #5251, .T. ) ;
#32565=VECTOR ( 'NONE', #13637, 1000.000000000000000 ) ;
#32586=VERTEX_POINT ( 'NONE', #27446 ) ;
#32599=EDGE_LOOP ( 'NONE', ( #10005, #10436 ) ) ;
#32604=EDGE_CURVE ( 'NONE', #26363, #33969, #17171, .T. ) ;
#32632=VECTOR ( 'NONE', #3680, 1000.000000000000000 ) ;
#32651=EDGE_CURVE ( 'NONE', #10949, #22703, #26425, .T. ) ;
#32672=DIRECTION ( 'NONE',  ( 1.000000000000000000, 0.000000000000000000, 0.000000000000000000 ) ) ;
#32686=AXIS2_PLACEMENT_3D ( 'NONE', #26225, #7134, #28751 ) ;
#32690=VERTEX_POINT ( 'NONE', #23397 ) ;
#32694=CARTESIAN_POINT ( 'NONE',  ( -50.00000000000000000, 6.123233995736780087E-16, 5.000000000000011546 ) ) ;
#32710=CIRCLE ( 'NONE', #7980, 7.999999999999992895 ) ;
#32712=FACE_BOUND ( 'NONE', #32599, .T. ) ;
#32723=DIRECTION ( 'NONE',  ( -1.000000000000000000, 0.000000000000000000, 0.000000000000000000 ) ) ;
#32724=DIRECTION ( 'NONE',  ( -1.000000000000000000, -0.000000000000000000, -0.000000000000000000 ) ) ;
#32732=CARTESIAN_POINT ( 'NONE',  ( 55.00000000000000000, -25.98076211353320275, 78.99999999999992895 ) ) ;
#32740=CARTESIAN_POINT ( 'NONE',  ( 50.00000000000000000, -25.98076211353320275, 84.99999999999992895 ) ) ;
#32745=EDGE_CURVE ( 'NONE', #10703, #10849, #34396, .T. ) ;
#32754=CARTESIAN_POINT ( 'NONE',  ( -50.00000000000000000, 0.000000000000000000, 8.000000000000000000 ) ) ;
#32780=EDGE_CURVE ( 'NONE', #19260, #34014, #15451, .T. ) ;
#32790=ORIENTED_EDGE ( 'NONE', *, *, #28887, .F. ) ;
#32821=EDGE_LOOP ( 'NONE', ( #15320, #28125, #12642, #25475 ) ) ;
#32833=CIRCLE ( 'NONE', #2932, 5.000000000000011546 ) ;
#32884=CARTESIAN_POINT ( 'NONE',  ( 46.00000000000000000, 0.000000000000000000, 70.00000000000000000 ) ) ;
#32888=PLANE ( 'NONE',  #20882 ) ;
#32925=DIRECTION ( 'NONE',  ( 0.000000000000000000, 0.000000000000000000, 1.000000000000000000 ) ) ;
#32944=CARTESIAN_POINT ( 'NONE',  ( -50.00000000000000000, 19.99999999999998934, 120.0000000000000000 ) ) ;
#32953=DIRECTION ( 'NONE',  ( 0.000000000000000000, 0.000000000000000000, 1.000000000000000000 ) ) ;
#32964=VERTEX_POINT ( 'NONE', #13146 ) ;
#32968=EDGE_CURVE ( 'NONE', #24250, #21944, #3449, .T. ) ;
#33007=VERTEX_POINT ( 'NONE', #19405 ) ;
#33034=DIRECTION ( 'NONE',  ( -1.000000000000000000, 0.000000000000000000, -0.000000000000000000 ) ) ;
#33041=DIRECTION ( 'NONE',  ( -0.000000000000000000, 0.000000000000000000, 1.000000000000000000 ) ) ;
#33052=( NAMED_UNIT ( * ) PLANE_ANGLE_UNIT ( ) SI_UNIT ( $, .RADIAN. ) );
#33066=CARTESIAN_POINT ( 'NONE',  ( 50.00000000000000000, 10.00000000000000888, -15.00000000000000178 ) ) ;
#33073=CARTESIAN_POINT ( 'NONE',  ( 50.00000000000000711, -25.98076211353320275, 84.99999999999994316 ) ) ;
#33088=ORIENTED_EDGE ( 'NONE', *, *, #788, .T. ) ;
#33094=FACE_OUTER_BOUND ( 'NONE', #9414, .T. ) ;
#33098=ORIENTED_EDGE ( 'NONE', *, *, #23549, .T. ) ;
#33100=DIRECTION ( 'NONE',  ( 0.000000000000000000, 0.000000000000000000, -1.000000000000000000 ) ) ;
#33130=ORIENTED_EDGE ( 'NONE', *, *, #33806, .F. ) ;
#33150=CYLINDRICAL_SURFACE ( 'NONE', #11375, 6.000000000000005329 ) ;
#33163=VECTOR ( 'NONE', #8080, 1000.000000000000000 ) ;
#33169=CARTESIAN_POINT ( 'NONE',  ( 0.000000000000000000, 0.000000000000000000, -25.00000000000000000 ) ) ;
#33174=VERTEX_POINT ( 'NONE', #21873 ) ;
#33189=VECTOR ( 'NONE', #27639, 1000.000000000000000 ) ;
#33195=VECTOR ( 'NONE', #26237, 1000.000000000000000 ) ;
#33196=CIRCLE ( 'NONE', #4485, 11.00000000000001066 ) ;
#33200=DIRECTION ( 'NONE',  ( -1.000000000000000000, 0.000000000000000000, -0.000000000000000000 ) ) ;
#33203=AXIS2_PLACEMENT_3D ( 'NONE', #35263, #32724, #21537 ) ;
#33205=DIRECTION ( 'NONE',  ( 0.000000000000000000, -1.000000000000000000, 0.000000000000000000 ) ) ;
#33215=DIRECTION ( 'NONE',  ( 0.000000000000000000, 0.000000000000000000, 1.000000000000000000 ) ) ;
#33221=CARTESIAN_POINT ( 'NONE',  ( 50.00000000000000711, 0.000000000000000000, 70.00000000000000000 ) ) ;
#33231=VECTOR ( 'NONE', #17783, 1000.000000000000000 ) ;
#33234=CARTESIAN_POINT ( 'NONE',  ( -50.00000000000000000, 0.000000000000000000, 11.00000000000000000 ) ) ;
#33246=AXIS2_PLACEMENT_3D ( 'NONE', #13968, #30014, #28014 ) ;
#33266=CARTESIAN_POINT ( 'NONE',  ( -29.99999999999999645, -26.99999999999999645, 113.9999999999999858 ) ) ;
#33280=FACE_OUTER_BOUND ( 'NONE', #22055, .T. ) ;
#33286=EDGE_CURVE ( 'NONE', #33174, #26283, #19679, .T. ) ;
#33312=CARTESIAN_POINT ( 'NONE',  ( 50.00000000000000000, 0.000000000000000000, -11.00000000000000000 ) ) ;
#33326=EDGE_CURVE ( 'NONE', #16219, #24282, #11947, .T. ) ;
#33343=DIRECTION ( 'NONE',  ( -1.000000000000000000, -1.734723475976807094E-16, 0.000000000000000000 ) ) ;
#33357=DIRECTION ( 'NONE',  ( 0.000000000000000000, 0.000000000000000000, -1.000000000000000000 ) ) ;
#33363=DIRECTION ( 'NONE',  ( 0.000000000000000000, 0.000000000000000000, -1.000000000000000000 ) ) ;
#33374=CARTESIAN_POINT ( 'NONE',  ( -29.99999999999999645, -26.99999999999999645, 113.9999999999999858 ) ) ;
#33384=DIRECTION ( 'NONE',  ( -1.000000000000000000, 0.000000000000000000, -0.000000000000000000 ) ) ;
#33395=EDGE_CURVE ( 'NONE', #35062, #17795, #23438, .T. ) ;
#33414=DIRECTION ( 'NONE',  ( -1.000000000000000000, -0.000000000000000000, -0.000000000000000000 ) ) ;
#33422=EDGE_CURVE ( 'NONE', #19029, #17673, #11360, .T. ) ;
#33442=CIRCLE ( 'NONE', #17916, 10.99999999999999645 ) ;
#33466=VERTEX_POINT ( 'NONE', #18905 ) ;
#33483=ORIENTED_EDGE ( 'NONE', *, *, #15129, .F. ) ;
#33533=LINE ( 'NONE', #33709, #528 ) ;
#33534=VECTOR ( 'NONE', #18876, 1000.000000000000000 ) ;
#33537=CARTESIAN_POINT ( 'NONE',  ( -55.00000000000000000, -25.98076211353320275, 78.99999999999992895 ) ) ;
#33558=ORIENTED_EDGE ( 'NONE', *, *, #34346, .T. ) ;
#33573=PLANE ( 'NONE',  #18408 ) ;
#33582=CARTESIAN_POINT ( 'NONE',  ( 46.00000000000000000, -25.98076211353320275, 95.99999999999991473 ) ) ;
#33598=DIRECTION ( 'NONE',  ( -1.000000000000000000, 0.000000000000000000, 0.000000000000000000 ) ) ;
#33604=CARTESIAN_POINT ( 'NONE',  ( 0.000000000000000000, 10.00000000000000888, -15.00000000000000178 ) ) ;
#33616=AXIS2_PLACEMENT_3D ( 'NONE', #15429, #26442, #21200 ) ;
#33645=VERTEX_POINT ( 'NONE', #25020 ) ;
#33653=ORIENTED_EDGE ( 'NONE', *, *, #30688, .T. ) ;
#33662=DIRECTION ( 'NONE',  ( -0.000000000000000000, -0.000000000000000000, -1.000000000000000000 ) ) ;
#33687=EDGE_CURVE ( 'NONE', #18294, #26363, #873, .T. ) ;
#33706=ORIENTED_EDGE ( 'NONE', *, *, #14899, .F. ) ;
#33708=AXIS2_PLACEMENT_3D ( 'NONE', #20749, #22926, #23279 ) ;
#33709=CARTESIAN_POINT ( 'NONE',  ( -49.99999999999998579, -60.00000000000000000, 120.0000000000000000 ) ) ;
#33733=CARTESIAN_POINT ( 'NONE',  ( -55.00000000000000000, 6.123233995736780087E-16, 5.000000000000011546 ) ) ;
#33754=DIRECTION ( 'NONE',  ( 0.000000000000000000, 0.000000000000000000, -1.000000000000000000 ) ) ;
#33777=LINE ( 'NONE', #25322, #7284 ) ;
#33790=EDGE_LOOP ( 'NONE', ( #27552, #16058, #29825, #14411 ) ) ;
#33801=PRODUCT_CONTEXT ( 'NONE', #3670, 'mechanical' ) ;
#33806=EDGE_CURVE ( 'NONE', #13387, #4303, #9866, .T. ) ;
#33844=ORIENTED_EDGE ( 'NONE', *, *, #8594, .F. ) ;
#33847=EDGE_CURVE ( 'NONE', #19260, #2874, #35560, .T. ) ;
#33860=CARTESIAN_POINT ( 'NONE',  ( -46.00000000000000000, 0.000000000000000000, 0.000000000000000000 ) ) ;
#33867=VERTEX_POINT ( 'NONE', #12222 ) ;
#33872=ORIENTED_EDGE ( 'NONE', *, *, #20697, .T. ) ;
#33879=FACE_BOUND ( 'NONE', #23556, .T. ) ;
#33892=EDGE_CURVE ( 'NONE', #17467, #30036, #6777, .T. ) ;
#33899=CARTESIAN_POINT ( 'NONE',  ( -55.00000000000000000, -25.98076211353320275, 90.99999999999994316 ) ) ;
#33914=CARTESIAN_POINT ( 'NONE',  ( -46.00000000000000000, 0.000000000000000000, 11.00000000000000000 ) ) ;
#33919=DIRECTION ( 'NONE',  ( 1.000000000000000000, 1.387778780781445922E-16, 0.000000000000000000 ) ) ;
#33925=PRODUCT_DEFINITION ( 'UNKNOWN', '', #21264, #11217 ) ;
#33936=EDGE_CURVE ( 'NONE', #20350, #18294, #481, .T. ) ;
#33967=ORIENTED_EDGE ( 'NONE', *, *, #12761, .T. ) ;
#33969=VERTEX_POINT ( 'NONE', #31622 ) ;
#33973=CARTESIAN_POINT ( 'NONE',  ( 55.00000000000000000, 0.000000000000000000, 70.00000000000000000 ) ) ;
#33997=CARTESIAN_POINT ( 'NONE',  ( 46.00000000000000000, 1.347111479062088405E-15, 11.00000000000000000 ) ) ;
#34001=AXIS2_PLACEMENT_3D ( 'NONE', #29517, #26996, #26459 ) ;
#34014=VERTEX_POINT ( 'NONE', #14499 ) ;
#34015=EDGE_CURVE ( 'NONE', #35000, #12018, #17716, .T. ) ;
#34027=EDGE_LOOP ( 'NONE', ( #20004, #6828 ) ) ;
#34052=EDGE_CURVE ( 'NONE', #17665, #32586, #22318, .T. ) ;
#34059=FACE_OUTER_BOUND ( 'NONE', #611, .T. ) ;
#34154=EDGE_CURVE ( 'NONE', #28784, #30634, #9118, .T. ) ;
#34157=FACE_OUTER_BOUND ( 'NONE', #9554, .T. ) ;
#34162=AXIS2_PLACEMENT_3D ( 'NONE', #22198, #33200, #3494 ) ;
#34176=EDGE_CURVE ( 'NONE', #17487, #15308, #15988, .T. ) ;
#34187=DIRECTION ( 'NONE',  ( 0.000000000000000000, 0.000000000000000000, -1.000000000000000000 ) ) ;
#34213=LINE ( 'NONE', #3797, #26053 ) ;
#34262=CARTESIAN_POINT ( 'NONE',  ( -46.00000000000000000, 0.000000000000000000, 70.00000000000000000 ) ) ;
#34263=EDGE_CURVE ( 'NONE', #28580, #35006, #15342, .T. ) ;
#34333=DIRECTION ( 'NONE',  ( 1.000000000000000000, -0.000000000000000000, 0.000000000000000000 ) ) ;
#34346=EDGE_CURVE ( 'NONE', #4839, #11168, #22829, .T. ) ;
#34347=ORIENTED_EDGE ( 'NONE', *, *, #33395, .T. ) ;
#34382=CARTESIAN_POINT ( 'NONE',  ( -55.00000000000000000, 0.000000000000000000, 0.000000000000000000 ) ) ;
#34396=LINE ( 'NONE', #14919, #4595 ) ;
#34420=ORIENTED_EDGE ( 'NONE', *, *, #17566, .F. ) ;
#34453=DIRECTION ( 'NONE',  ( 0.000000000000000000, 0.000000000000000000, 1.000000000000000000 ) ) ;
#34497=CARTESIAN_POINT ( 'NONE',  ( -55.00000000000000000, -2.775557561562891351E-14, 110.0000000000000000 ) ) ;
#34514=DIRECTION ( 'NONE',  ( 0.000000000000000000, 0.000000000000000000, 1.000000000000000000 ) ) ;
#34516=ADVANCED_FACE ( 'NONE', ( #6201, #2823 ), #441, .F. ) ;
#34539=CYLINDRICAL_SURFACE ( 'NONE', #35468, 10.99999999999999645 ) ;
#34569=ORIENTED_EDGE ( 'NONE', *, *, #21435, .F. ) ;
#34578=EDGE_CURVE ( 'NONE', #31888, #23379, #14143, .T. ) ;
#34586=ORIENTED_EDGE ( 'NONE', *, *, #7647, .F. ) ;
#34588=CARTESIAN_POINT ( 'NONE',  ( -49.99999999999998579, -60.00000000000000000, -25.00000000000000000 ) ) ;
#34597=ADVANCED_FACE ( 'NONE', ( #23473 ), #12131, .T. ) ;
#34706=CARTESIAN_POINT ( 'NONE',  ( -55.00000000000000000, 0.000000000000000000, 0.000000000000000000 ) ) ;
#34718=CARTESIAN_POINT ( 'NONE',  ( -49.99999999999999289, -25.98076211353320275, 90.99999999999994316 ) ) ;
#34775=CARTESIAN_POINT ( 'NONE',  ( 46.00000000000000000, 0.000000000000000000, 0.000000000000000000 ) ) ;
#34782=DIRECTION ( 'NONE',  ( 1.000000000000000000, 1.734723475976807094E-16, -0.000000000000000000 ) ) ;
#34859=LINE ( 'NONE', #35048, #23616 ) ;
#34864=DIRECTION ( 'NONE',  ( 1.000000000000000000, 0.000000000000000000, -0.000000000000000000 ) ) ;
#34887=CARTESIAN_POINT ( 'NONE',  ( -50.00000000000000000, -2.775557561562891351E-14, 110.0000000000000000 ) ) ;
#34900=DIRECTION ( 'NONE',  ( 1.000000000000000000, -0.000000000000000000, -0.000000000000000000 ) ) ;
#34905=AXIS2_PLACEMENT_3D ( 'NONE', #12802, #15477, #10584 ) ;
#34920=AXIS2_PLACEMENT_3D ( 'NONE', #31706, #4184, #19990 ) ;
#34966=AXIS2_PLACEMENT_3D ( 'NONE', #25028, #16560, #27568 ) ;
#34972=ORIENTED_EDGE ( 'NONE', *, *, #23648, .T. ) ;
#35000=VERTEX_POINT ( 'NONE', #13908 ) ;
#35003=CARTESIAN_POINT ( 'NONE',  ( 46.00000000000000000, 0.000000000000000000, -8.000000000000000000 ) ) ;
#35006=VERTEX_POINT ( 'NONE', #22000 ) ;
#35023=ADVANCED_FACE ( 'NONE', ( #5982 ), #22528, .F. ) ;
#35029=FACE_OUTER_BOUND ( 'NONE', #1562, .T. ) ;
#35048=CARTESIAN_POINT ( 'NONE',  ( -55.00000000000000000, 19.99999999999998934, 120.0000000000000000 ) ) ;
#35062=VERTEX_POINT ( 'NONE', #1654 ) ;
#35098=ADVANCED_FACE ( 'NONE', ( #9744, #33879, #28834, #26320, #34059 ), #14596, .T. ) ;
#35123=CARTESIAN_POINT ( 'NONE',  ( 50.00000000000000711, 0.000000000000000000, 0.000000000000000000 ) ) ;
#35140=VERTEX_POINT ( 'NONE', #9384 ) ;
#35147=AXIS2_PLACEMENT_3D ( 'NONE', #2053, #29942, #8500 ) ;
#35168=AXIS2_PLACEMENT_3D ( 'NONE', #29004, #20338, #12627 ) ;
#35174=EDGE_LOOP ( 'NONE', ( #19975, #17334, #12666, #205 ) ) ;
#35206=ORIENTED_EDGE ( 'NONE', *, *, #13439, .F. ) ;
#35220=DIRECTION ( 'NONE',  ( 1.000000000000000000, -0.000000000000000000, -0.000000000000000000 ) ) ;
#35231=VECTOR ( 'NONE', #23860, 1000.000000000000000 ) ;
#35251=DIRECTION ( 'NONE',  ( 0.000000000000000000, 0.000000000000000000, 1.000000000000000000 ) ) ;
#35263=CARTESIAN_POINT ( 'NONE',  ( -50.00000000000000000, 0.000000000000000000, 70.00000000000000000 ) ) ;
#35281=CIRCLE ( 'NONE', #18580, 6.000000000000005329 ) ;
#35288=LINE ( 'NONE', #10437, #8584 ) ;
#35302=ORIENTED_EDGE ( 'NONE', *, *, #20991, .F. ) ;
#35329=ADVANCED_FACE ( 'NONE', ( #12812 ), #18909, .T. ) ;
#35379=CARTESIAN_POINT ( 'NONE',  ( -49.99999999999999289, -25.98076211353320275, 84.99999999999992895 ) ) ;
#35386=AXIS2_PLACEMENT_3D ( 'NONE', #23678, #28905, #26200 ) ;
#35431=FACE_OUTER_BOUND ( 'NONE', #6673, .T. ) ;
#35454=CARTESIAN_POINT ( 'NONE',  ( -55.00000000000000000, -2.726571689596996976E-14, 114.0000000000000000 ) ) ;
#35468=AXIS2_PLACEMENT_3D ( 'NONE', #29139, #7864, #7683 ) ;
#35480=EDGE_CURVE ( 'NONE', #22703, #10949, #3475, .T. ) ;
#35481=VECTOR ( 'NONE', #12886, 1000.000000000000000 ) ;
#35499=DIRECTION ( 'NONE',  ( 0.000000000000000000, 0.000000000000000000, -1.000000000000000000 ) ) ;
#35505=AXIS2_PLACEMENT_3D ( 'NONE', #15564, #29285, #7125 ) ;
#35531=FACE_OUTER_BOUND ( 'NONE', #31346, .T. ) ;
#35534=AXIS2_PLACEMENT_3D ( 'NONE', #443, #20036, #28340 ) ;
#35540=ORIENTED_EDGE ( 'NONE', *, *, #20991, .T. ) ;
#35560=CIRCLE ( 'NONE', #19420, 7.999999999999992895 ) ;
#35571=EDGE_CURVE ( 'NONE', #16323, #32690, #4104, .T. ) ;
#35589=ORIENTED_EDGE ( 'NONE', *, *, #7535, .T. ) ;
#35601=DIRECTION ( 'NONE',  ( 1.000000000000000000, 0.000000000000000000, -0.000000000000000000 ) ) ;
ENDSEC;
END-ISO-10303-21;
